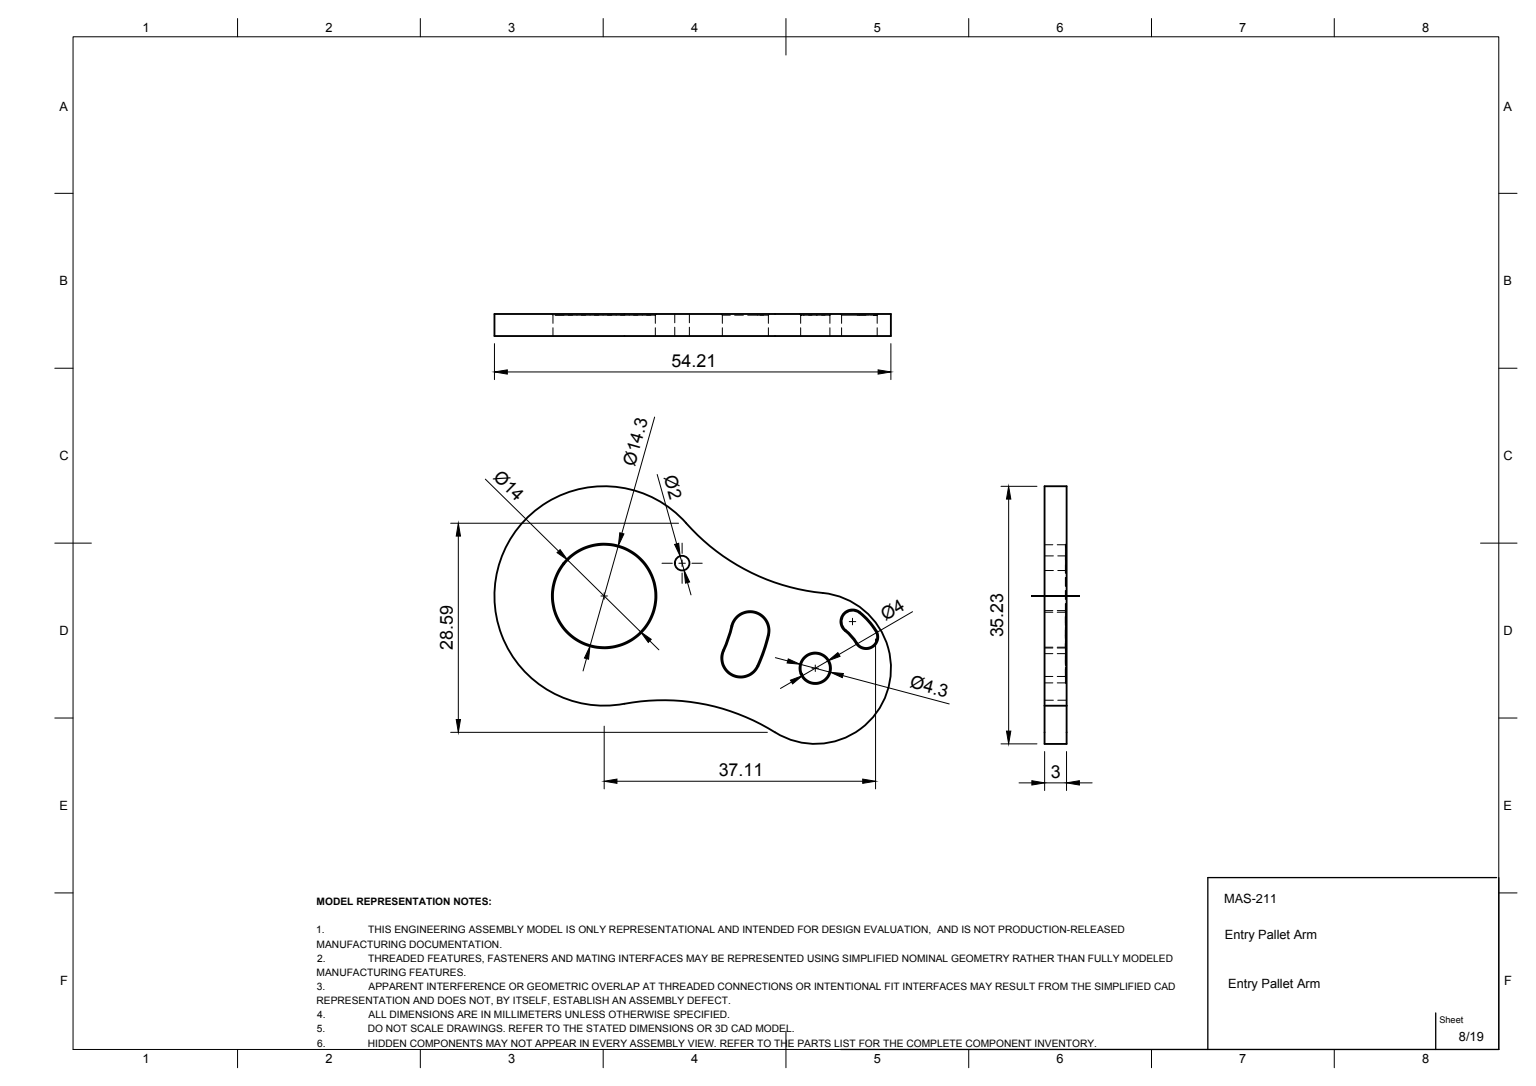
ISO-10303-21;
HEADER;
FILE_DESCRIPTION(
 (''),
 '2;1');
FILE_NAME ( 'Entry Pallet Arm.step', '2026-10-05T20:07:59+06:00', ( '' ), ( '' ), 'STEP AP214', 'Unspecified', '' );
FILE_SCHEMA (('AUTOMOTIVE_DESIGN { 1 0 10303 214 3 1 1 }'));
ENDSEC;
DATA;
#10=MECHANICAL_DESIGN_GEOMETRIC_PRESENTATION_REPRESENTATION('',(#325),#196741);
#131=ELLIPSE('',#8872,15.4840898363667,13.4083590367118) ;
#132=ELLIPSE('',#8873,20.0777465510975,17.3862071407653) ;
#133=ELLIPSE('',#8874,8.52758831083714,7.38294286669008) ;
#134=ELLIPSE('',#8875,5.66235728936404,4.9022943840305) ;
#325=STYLED_ITEM('',(#196765),#344) ;
#344=MANIFOLD_SOLID_BREP('Entry Pallet Arm',#8721) ;
#385=PLANE('',#8860) ;
#386=PLANE('',#8871) ;
#566=FACE_BOUND('',#1445,.T.) ;
#567=FACE_BOUND('',#1446,.T.) ;
#568=FACE_BOUND('',#1447,.T.) ;
#569=FACE_BOUND('',#1448,.T.) ;
#570=FACE_BOUND('',#1449,.T.) ;
#571=FACE_BOUND('',#1451,.T.) ;
#572=FACE_BOUND('',#1452,.T.) ;
#573=FACE_BOUND('',#1453,.T.) ;
#574=FACE_BOUND('',#1454,.T.) ;
#575=FACE_BOUND('',#1455,.T.) ;
#639=CIRCLE('',#8846,28.7407375552552) ;
#640=CIRCLE('',#8847,28.7407375552552) ;
#641=CIRCLE('',#8849,15.) ;
#642=CIRCLE('',#8850,15.) ;
#643=CIRCLE('',#8852,28.7407375552563) ;
#644=CIRCLE('',#8853,28.7407375552563) ;
#645=CIRCLE('',#8855,10.3432265401781) ;
#646=CIRCLE('',#8856,10.3432265401781) ;
#647=CIRCLE('',#8858,1.00000000000001) ;
#648=CIRCLE('',#8859,1.00000000000001) ;
#649=CIRCLE('',#8861,2.) ;
#650=CIRCLE('',#8862,23.0149881946395) ;
#651=CIRCLE('',#8863,2.4999999999999) ;
#652=CIRCLE('',#8864,18.0149881946822) ;
#653=CIRCLE('',#8865,2.49999999999983) ;
#654=CIRCLE('',#8866,7.00000000000001) ;
#655=CIRCLE('',#8867,1.50000000000001) ;
#656=CIRCLE('',#8868,6.6716132701064) ;
#657=CIRCLE('',#8869,1.49999999999977) ;
#658=CIRCLE('',#8870,9.6716132700902) ;
#659=CIRCLE('',#8877,2.00000000000002) ;
#660=CIRCLE('',#8880,18.0149881946813) ;
#661=CIRCLE('',#8884,7.00000000000001) ;
#662=CIRCLE('',#8887,1.49999999999978) ;
#663=CIRCLE('',#8889,6.6716132701049) ;
#836=B_SPLINE_SURFACE_WITH_KNOTS('',3,1,((#113116,#113117),(#113118,#113119),
(#113120,#113121),(#113122,#113123),(#113124,#113125),(#113126,#113127),
(#113128,#113129),(#113130,#113131),(#113132,#113133),(#113134,#113135),
(#113136,#113137),(#113138,#113139),(#113140,#113141),(#113142,#113143),
(#113144,#113145),(#113146,#113147),(#113148,#113149),(#113150,#113151),
(#113152,#113153)),.UNSPECIFIED.,.T.,.F.,.F.,(4,1,1,1,1,1,1,1,1,1,1,1,1,
1,1,1,4),(2,2),(0.,0.84428169467316,1.68856338934632,2.53284508400807,3.37712677866981,
4.22140847333581,5.06569016800181,5.90997186266355,6.75425355732529,7.5985352519836,
8.44281694664192,9.28709864130792,10.1313803359739,10.9756620306322,11.8199437252905,
12.664225419956,13.5085071146214),(-0.0112712723153948,0.214916064351503),
 .UNSPECIFIED.) ;
#837=B_SPLINE_SURFACE_WITH_KNOTS('',3,1,((#113155,#113156),(#113157,#113158),
(#113159,#113160),(#113161,#113162),(#113163,#113164),(#113165,#113166),
(#113167,#113168),(#113169,#113170),(#113171,#113172),(#113173,#113174),
(#113175,#113176)),.UNSPECIFIED.,.F.,.F.,.F.,(4,1,1,1,1,1,1,1,4),(2,2),
(0.,1.04064620349252,2.08129240698504,3.12193860703556,4.16258480708607,
5.2032310071414,6.24387720719673,7.28452341068926,8.32516961418179),(0.,
0.214915892336475),.UNSPECIFIED.) ;
#838=B_SPLINE_SURFACE_WITH_KNOTS('',3,1,((#113179,#113180),(#113181,#113182),
(#113183,#113184),(#113185,#113186)),.UNSPECIFIED.,.F.,.F.,.F.,(4,4),(2,
2),(-1.11022302462516E-16,3.4846841528001),(0.,0.212356567860224),
 .UNSPECIFIED.) ;
#839=B_SPLINE_SURFACE_WITH_KNOTS('',3,1,((#113188,#113189),(#113190,#113191),
(#113192,#113193),(#113194,#113195),(#113196,#113197),(#113198,#113199),
(#113200,#113201),(#113202,#113203),(#113204,#113205),(#113206,#113207),
(#113208,#113209)),.UNSPECIFIED.,.F.,.F.,.F.,(4,1,1,1,1,1,1,1,4),(2,2),
(0.,1.04062614942685,2.0812522988537,3.12187844827608,4.16250459769846,
5.20313074711661,6.24375689653477,7.28438304596783,8.32500919540089),(0.,
0.214916063344347),.UNSPECIFIED.) ;
#840=B_SPLINE_SURFACE_WITH_KNOTS('',3,1,((#113211,#113212),(#113213,#113214),
(#113215,#113216),(#113217,#113218)),.UNSPECIFIED.,.F.,.F.,.F.,(4,4),(2,
2),(1.11022302462516E-16,4.51848390029441),(-6.99189760998493E-5,0.212356567829038),
 .UNSPECIFIED.) ;
#841=B_SPLINE_SURFACE_WITH_KNOTS('',3,1,((#113219,#113220),(#113221,#113222),
(#113223,#113224),(#113225,#113226),(#113227,#113228),(#113229,#113230),
(#113231,#113232),(#113233,#113234),(#113235,#113236),(#113237,#113238),
(#113239,#113240),(#113241,#113242),(#113243,#113244),(#113245,#113246),
(#113247,#113248),(#113249,#113250),(#113251,#113252),(#113253,#113254),
(#113255,#113256)),.UNSPECIFIED.,.T.,.F.,.F.,(4,1,1,1,1,1,1,1,1,1,1,1,1,
1,1,1,4),(2,2),(0.,2.69519445779221,5.61545499238393,8.53571552697323,11.2309099847624,
13.9261044425515,16.8463649771433,19.7666255117326,22.4618199695218,25.1570144273109,
28.0772749619002,30.9975354964919,33.6927299542811,36.3879244120703,39.3081849466596,
42.2284454812513,44.9236399390405),(-0.021515064961137,0.21515064961137),
 .UNSPECIFIED.) ;
#842=B_SPLINE_SURFACE_WITH_KNOTS('',3,1,((#113258,#113259),(#113260,#113261),
(#113262,#113263),(#113264,#113265)),.UNSPECIFIED.,.F.,.F.,.F.,(4,4),(2,
2),(0.,3.40704145701401),(-0.000292126274588819,0.212844506430303),
 .UNSPECIFIED.) ;
#843=B_SPLINE_SURFACE_WITH_KNOTS('',3,1,((#113268,#113269),(#113270,#113271),
(#113272,#113273),(#113274,#113275),(#113276,#113277),(#113278,#113279),
(#113280,#113281),(#113282,#113283),(#113284,#113285)),.UNSPECIFIED.,.F.,
 .F.,.F.,(4,1,1,1,1,1,4),(2,2),(-0.00583358110187113,1.29587390932424,1.94381087119108,
2.59174783305793,3.23968479492214,3.88762175678635,5.18932922796654),(-0.00583356183498457,
0.218727515757821),.UNSPECIFIED.) ;
#844=B_SPLINE_SURFACE_WITH_KNOTS('',3,1,((#113287,#113288),(#113289,#113290),
(#113291,#113292),(#113293,#113294)),.UNSPECIFIED.,.F.,.F.,.F.,(4,4),(2,
2),(0.,2.26229870547718),(0.,0.212844507129699),.UNSPECIFIED.) ;
#845=B_SPLINE_SURFACE_WITH_KNOTS('',3,1,((#113296,#113297),(#113298,#113299),
(#113300,#113301),(#113302,#113303),(#113304,#113305),(#113306,#113307),
(#113308,#113309),(#113310,#113311),(#113312,#113313)),.UNSPECIFIED.,.F.,
 .F.,.F.,(4,1,1,1,1,1,4),(2,2),(0.,1.29587422179682,1.94381133989722,2.59174845799762,
3.23968557610065,3.88762269420369,5.18349660704779),(0.,0.218727518540508),
 .UNSPECIFIED.) ;
#954=FACE_OUTER_BOUND('',#1439,.T.) ;
#955=FACE_OUTER_BOUND('',#1440,.T.) ;
#956=FACE_OUTER_BOUND('',#1441,.T.) ;
#957=FACE_OUTER_BOUND('',#1442,.T.) ;
#958=FACE_OUTER_BOUND('',#1443,.T.) ;
#959=FACE_OUTER_BOUND('',#1444,.T.) ;
#960=FACE_OUTER_BOUND('',#1450,.T.) ;
#961=FACE_OUTER_BOUND('',#1456,.T.) ;
#962=FACE_OUTER_BOUND('',#1457,.T.) ;
#963=FACE_OUTER_BOUND('',#1458,.T.) ;
#964=FACE_OUTER_BOUND('',#1459,.T.) ;
#965=FACE_OUTER_BOUND('',#1460,.T.) ;
#966=FACE_OUTER_BOUND('',#1461,.T.) ;
#967=FACE_OUTER_BOUND('',#1462,.T.) ;
#968=FACE_OUTER_BOUND('',#1463,.T.) ;
#969=FACE_OUTER_BOUND('',#1464,.T.) ;
#970=FACE_OUTER_BOUND('',#1465,.T.) ;
#971=FACE_OUTER_BOUND('',#1466,.T.) ;
#972=FACE_OUTER_BOUND('',#1467,.T.) ;
#973=FACE_OUTER_BOUND('',#1468,.T.) ;
#974=FACE_OUTER_BOUND('',#1469,.T.) ;
#975=FACE_OUTER_BOUND('',#1470,.T.) ;
#976=FACE_OUTER_BOUND('',#1471,.T.) ;
#977=FACE_OUTER_BOUND('',#1472,.T.) ;
#978=FACE_OUTER_BOUND('',#1473,.T.) ;
#979=FACE_OUTER_BOUND('',#1474,.T.) ;
#980=FACE_OUTER_BOUND('',#1475,.T.) ;
#1439=EDGE_LOOP('',(#6086,#6087,#6088,#6089)) ;
#1440=EDGE_LOOP('',(#6090,#6091,#6092,#6093)) ;
#1441=EDGE_LOOP('',(#6094,#6095,#6096,#6097)) ;
#1442=EDGE_LOOP('',(#6098,#6099,#6100,#6101)) ;
#1443=EDGE_LOOP('',(#6102,#6103,#6104,#6105)) ;
#1444=EDGE_LOOP('',(#6106,#6107,#6108,#6109)) ;
#1445=EDGE_LOOP('',(#6110)) ;
#1446=EDGE_LOOP('',(#6111,#6112,#6113,#6114)) ;
#1447=EDGE_LOOP('',(#6115)) ;
#1448=EDGE_LOOP('',(#6116,#6117,#6118,#6119)) ;
#1449=EDGE_LOOP('',(#6120)) ;
#1450=EDGE_LOOP('',(#6121,#6122,#6123,#6124)) ;
#1451=EDGE_LOOP('',(#6125)) ;
#1452=EDGE_LOOP('',(#6126)) ;
#1453=EDGE_LOOP('',(#6127,#6128,#6129,#6130)) ;
#1454=EDGE_LOOP('',(#6131,#6132,#6133,#6134)) ;
#1455=EDGE_LOOP('',(#6135)) ;
#1456=EDGE_LOOP('',(#6136,#6137,#6138,#6139)) ;
#1457=EDGE_LOOP('',(#6140,#6141,#6142,#6143)) ;
#1458=EDGE_LOOP('',(#6144,#6145,#6146,#6147)) ;
#1459=EDGE_LOOP('',(#6148,#6149,#6150,#6151)) ;
#1460=EDGE_LOOP('',(#6152,#6153,#6154,#6155)) ;
#1461=EDGE_LOOP('',(#6156,#6157,#6158,#6159)) ;
#1462=EDGE_LOOP('',(#6160,#6161,#6162,#6163)) ;
#1463=EDGE_LOOP('',(#6164,#6165,#6166,#6167)) ;
#1464=EDGE_LOOP('',(#6168,#6169,#6170,#6171)) ;
#1465=EDGE_LOOP('',(#6172,#6173,#6174,#6175)) ;
#1466=EDGE_LOOP('',(#6176,#6177,#6178,#6179)) ;
#1467=EDGE_LOOP('',(#6180,#6181,#6182,#6183)) ;
#1468=EDGE_LOOP('',(#6184,#6185,#6186,#6187)) ;
#1469=EDGE_LOOP('',(#6188,#6189,#6190,#6191)) ;
#1470=EDGE_LOOP('',(#6192,#6193,#6194,#6195)) ;
#1471=EDGE_LOOP('',(#6196,#6197,#6198,#6199)) ;
#1472=EDGE_LOOP('',(#6200,#6201,#6202,#6203)) ;
#1473=EDGE_LOOP('',(#6204,#6205,#6206,#6207)) ;
#1474=EDGE_LOOP('',(#6208,#6209,#6210,#6211)) ;
#1475=EDGE_LOOP('',(#6212,#6213,#6214,#6215)) ;
#1956=LINE('',#112886,#2659) ;
#1957=LINE('',#112889,#2660) ;
#1958=LINE('',#112894,#2661) ;
#1959=LINE('',#112900,#2662) ;
#1960=LINE('',#112909,#2663) ;
#1961=LINE('',#113041,#2664) ;
#1962=LINE('',#113044,#2665) ;
#1963=LINE('',#113046,#2666) ;
#1964=LINE('',#113060,#2667) ;
#1965=LINE('',#113064,#2668) ;
#1966=LINE('',#113086,#2669) ;
#1967=LINE('',#113089,#2670) ;
#1968=LINE('',#113091,#2671) ;
#1969=LINE('',#113100,#2672) ;
#1970=LINE('',#113104,#2673) ;
#1971=LINE('',#113154,#2674) ;
#1972=LINE('',#113177,#2675) ;
#1973=LINE('',#113178,#2676) ;
#1974=LINE('',#113187,#2677) ;
#1975=LINE('',#113210,#2678) ;
#1976=LINE('',#113257,#2679) ;
#1977=LINE('',#113266,#2680) ;
#1978=LINE('',#113267,#2681) ;
#1979=LINE('',#113286,#2682) ;
#1980=LINE('',#113295,#2683) ;
#2659=VECTOR('',#9750,10.) ;
#2660=VECTOR('',#9753,10.) ;
#2661=VECTOR('',#9758,10.) ;
#2662=VECTOR('',#9765,10.) ;
#2663=VECTOR('',#9778,1.00000000000001) ;
#2664=VECTOR('',#9817,2.00000000000002) ;
#2665=VECTOR('',#9820,10.) ;
#2666=VECTOR('',#9821,10.) ;
#2667=VECTOR('',#9824,10.) ;
#2668=VECTOR('',#9829,10.) ;
#2669=VECTOR('',#9836,6.99999999999997) ;
#2670=VECTOR('',#9839,10.) ;
#2671=VECTOR('',#9840,10.) ;
#2672=VECTOR('',#9843,10.) ;
#2673=VECTOR('',#9848,10.) ;
#2674=VECTOR('',#9853,10.) ;
#2675=VECTOR('',#9854,10.) ;
#2676=VECTOR('',#9855,10.) ;
#2677=VECTOR('',#9856,10.) ;
#2678=VECTOR('',#9857,10.) ;
#2679=VECTOR('',#9858,10.) ;
#2680=VECTOR('',#9859,10.) ;
#2681=VECTOR('',#9860,10.) ;
#2682=VECTOR('',#9861,10.) ;
#2683=VECTOR('',#9862,10.) ;
#3408=B_SPLINE_CURVE_WITH_KNOTS('',3,(#112934,#112935,#112936,#112937,#112938,
#112939,#112940,#112941,#112942,#112943,#112944,#112945,#112946,#112947,
#112948,#112949,#112950,#112951,#112952),.UNSPECIFIED.,.T.,.F.,(4,1,1,1,
1,1,1,1,1,1,1,1,1,1,1,1,4),(0.,2.69519445779221,5.61545499238393,8.53571552697323,
11.2309099847624,13.9261044425515,16.8463649771433,19.7666255117326,22.4618199695218,
25.1570144273109,28.0772749619002,30.9975354964919,33.6927299542811,36.3879244120703,
39.3081849466596,42.2284454812513,44.9236399390405),.UNSPECIFIED.) ;
#3409=B_SPLINE_CURVE_WITH_KNOTS('',3,(#112955,#112956,#112957,#112958,#112959,
#112960,#112961,#112962,#112963,#112964,#112965),.UNSPECIFIED.,.F.,.F.,
(4,1,1,1,1,1,1,1,4),(0.,1.04064620349252,2.08129240698504,3.12193860703556,
4.16258480708607,5.2032310071414,6.24387720719673,7.28452341068926,8.32516961418179),
 .UNSPECIFIED.) ;
#3410=B_SPLINE_CURVE_WITH_KNOTS('',3,(#112969,#112970,#112971,#112972,#112973,
#112974,#112975,#112976,#112977,#112978,#112979),.UNSPECIFIED.,.F.,.F.,
(4,1,1,1,1,1,1,1,4),(0.,1.04062614942685,2.0812522988537,3.12187844827608,
4.16250459769846,5.20313074711661,6.24375689653477,7.28438304596783,8.32500919540089),
 .UNSPECIFIED.) ;
#3411=B_SPLINE_CURVE_WITH_KNOTS('',3,(#112985,#112986,#112987,#112988,#112989,
#112990,#112991,#112992,#112993,#112994,#112995,#112996,#112997,#112998,
#112999,#113000,#113001,#113002,#113003,#113004,#113005,#113006),
 .UNSPECIFIED.,.F.,.F.,(4,2,2,2,2,2,2,2,2,2,4),(-0.482562577818028,-0.447777673419887,
-0.413036999106612,-0.354121907354326,-0.297189647078672,-0.24122658651999,
-0.185260249381691,-0.128411301285868,-0.0694119365245573,-0.0347286016619977,
0.),.UNSPECIFIED.) ;
#3412=B_SPLINE_CURVE_WITH_KNOTS('',3,(#113009,#113010,#113011,#113012,#113013,
#113014,#113015,#113016,#113017),.UNSPECIFIED.,.F.,.F.,(4,1,1,1,1,1,4),
(0.,1.29587422179682,1.94381133989722,2.59174845799762,3.23968557610065,
3.88762269420369,5.18349660704779),.UNSPECIFIED.) ;
#3413=B_SPLINE_CURVE_WITH_KNOTS('',3,(#113019,#113020,#113021,#113022,#113023,
#113024,#113025,#113026,#113027,#113028,#113029,#113030,#113031,#113032,
#113033,#113034,#113035,#113036,#113037),.UNSPECIFIED.,.T.,.F.,(4,1,1,1,
1,1,1,1,1,1,1,1,1,1,1,1,4),(0.,0.84428169467316,1.68856338934632,2.53284508400807,
3.37712677866981,4.22140847333581,5.06569016800181,5.90997186266355,6.75425355732529,
7.5985352519836,8.44281694664192,9.28709864130792,10.1313803359739,10.9756620306322,
11.8199437252905,12.664225419956,13.5085071146214),.UNSPECIFIED.) ;
#3414=B_SPLINE_CURVE_WITH_KNOTS('',3,(#113047,#113048,#113049,#113050,#113051,
#113052,#113053,#113054,#113055,#113056,#113057),.UNSPECIFIED.,.F.,.F.,
(4,1,1,1,1,1,1,1,4),(0.,1.04064620349252,2.08129240698504,3.12193860703556,
4.16258480708607,5.2032310071414,6.24387720719673,7.28452341068926,8.32516961418179),
 .UNSPECIFIED.) ;
#3415=B_SPLINE_CURVE_WITH_KNOTS('',3,(#113065,#113066,#113067,#113068,#113069,
#113070,#113071,#113072,#113073,#113074,#113075),.UNSPECIFIED.,.F.,.F.,
(4,1,1,1,1,1,1,1,4),(0.,1.04062614942685,2.0812522988537,3.12187844827608,
4.16250459769846,5.20313074711661,6.24375689653477,7.28438304596783,8.32500919540089),
 .UNSPECIFIED.) ;
#3416=B_SPLINE_CURVE_WITH_KNOTS('',3,(#113077,#113078,#113079,#113080,#113081,
#113082),.UNSPECIFIED.,.F.,.F.,(4,2,4),(0.,0.224505556318787,0.44901111263762),
 .UNSPECIFIED.) ;
#3417=B_SPLINE_CURVE_WITH_KNOTS('',3,(#113092,#113093,#113094,#113095,#113096,
#113097),.UNSPECIFIED.,.F.,.F.,(4,2,4),(6.6871801508411E-9,0.167853757777579,
0.335707403334044),.UNSPECIFIED.) ;
#3418=B_SPLINE_CURVE_WITH_KNOTS('',3,(#113107,#113108,#113109,#113110,#113111,
#113112,#113113,#113114,#113115),.UNSPECIFIED.,.F.,.F.,(4,1,1,1,1,1,4),
(1.11022302462516E-16,1.29587422179682,1.94381133989722,2.59174845799762,
3.23968557610065,3.88762269420369,5.18349660704779),.UNSPECIFIED.) ;
#3623=VERTEX_POINT('',#112882) ;
#3624=VERTEX_POINT('',#112883) ;
#3625=VERTEX_POINT('',#112885) ;
#3626=VERTEX_POINT('',#112887) ;
#3627=VERTEX_POINT('',#112891) ;
#3628=VERTEX_POINT('',#112893) ;
#3629=VERTEX_POINT('',#112897) ;
#3630=VERTEX_POINT('',#112899) ;
#3631=VERTEX_POINT('',#112906) ;
#3632=VERTEX_POINT('',#112908) ;
#3633=VERTEX_POINT('',#112912) ;
#3634=VERTEX_POINT('',#112914) ;
#3635=VERTEX_POINT('',#112915) ;
#3636=VERTEX_POINT('',#112917) ;
#3637=VERTEX_POINT('',#112919) ;
#3638=VERTEX_POINT('',#112922) ;
#3639=VERTEX_POINT('',#112924) ;
#3640=VERTEX_POINT('',#112925) ;
#3641=VERTEX_POINT('',#112927) ;
#3642=VERTEX_POINT('',#112929) ;
#3643=VERTEX_POINT('',#112933) ;
#3644=VERTEX_POINT('',#112953) ;
#3645=VERTEX_POINT('',#112954) ;
#3646=VERTEX_POINT('',#112966) ;
#3647=VERTEX_POINT('',#112968) ;
#3648=VERTEX_POINT('',#112981) ;
#3649=VERTEX_POINT('',#112982) ;
#3650=VERTEX_POINT('',#112984) ;
#3651=VERTEX_POINT('',#113007) ;
#3652=VERTEX_POINT('',#113018) ;
#3653=VERTEX_POINT('',#113039) ;
#3654=VERTEX_POINT('',#113043) ;
#3655=VERTEX_POINT('',#113045) ;
#3656=VERTEX_POINT('',#113059) ;
#3657=VERTEX_POINT('',#113063) ;
#3658=VERTEX_POINT('',#113084) ;
#3659=VERTEX_POINT('',#113088) ;
#3660=VERTEX_POINT('',#113090) ;
#3661=VERTEX_POINT('',#113099) ;
#3662=VERTEX_POINT('',#113103) ;
#4551=EDGE_CURVE('',#3623,#3624,#639,.T.) ;
#4552=EDGE_CURVE('',#3624,#3625,#1956,.T.) ;
#4553=EDGE_CURVE('',#3626,#3625,#640,.T.) ;
#4554=EDGE_CURVE('',#3623,#3626,#1957,.T.) ;
#4555=EDGE_CURVE('',#3624,#3627,#641,.T.) ;
#4556=EDGE_CURVE('',#3627,#3628,#1958,.T.) ;
#4557=EDGE_CURVE('',#3625,#3628,#642,.T.) ;
#4558=EDGE_CURVE('',#3627,#3629,#643,.T.) ;
#4559=EDGE_CURVE('',#3629,#3630,#1959,.T.) ;
#4560=EDGE_CURVE('',#3628,#3630,#644,.T.) ;
#4561=EDGE_CURVE('',#3629,#3623,#645,.T.) ;
#4562=EDGE_CURVE('',#3630,#3626,#646,.T.) ;
#4563=EDGE_CURVE('',#3631,#3631,#647,.T.) ;
#4564=EDGE_CURVE('',#3631,#3632,#1960,.T.) ;
#4565=EDGE_CURVE('',#3632,#3632,#648,.T.) ;
#4566=EDGE_CURVE('',#3633,#3633,#649,.T.) ;
#4567=EDGE_CURVE('',#3634,#3635,#650,.T.) ;
#4568=EDGE_CURVE('',#3636,#3634,#651,.T.) ;
#4569=EDGE_CURVE('',#3637,#3636,#652,.T.) ;
#4570=EDGE_CURVE('',#3635,#3637,#653,.T.) ;
#4571=EDGE_CURVE('',#3638,#3638,#654,.T.) ;
#4572=EDGE_CURVE('',#3639,#3640,#655,.T.) ;
#4573=EDGE_CURVE('',#3641,#3639,#656,.T.) ;
#4574=EDGE_CURVE('',#3642,#3641,#657,.T.) ;
#4575=EDGE_CURVE('',#3640,#3642,#658,.T.) ;
#4576=EDGE_CURVE('',#3643,#3643,#3408,.T.) ;
#4577=EDGE_CURVE('',#3644,#3645,#3409,.T.) ;
#4578=EDGE_CURVE('',#3645,#3646,#131,.T.) ;
#4579=EDGE_CURVE('',#3646,#3647,#3410,.T.) ;
#4580=EDGE_CURVE('',#3647,#3644,#132,.T.) ;
#4581=EDGE_CURVE('',#3648,#3649,#133,.T.) ;
#4582=EDGE_CURVE('',#3649,#3650,#3411,.T.) ;
#4583=EDGE_CURVE('',#3650,#3651,#134,.T.) ;
#4584=EDGE_CURVE('',#3651,#3648,#3412,.T.) ;
#4585=EDGE_CURVE('',#3652,#3652,#3413,.T.) ;
#4586=EDGE_CURVE('',#3653,#3653,#659,.T.) ;
#4587=EDGE_CURVE('',#3653,#3633,#1961,.T.) ;
#4588=EDGE_CURVE('',#3635,#3654,#1962,.T.) ;
#4589=EDGE_CURVE('',#3637,#3655,#1963,.T.) ;
#4590=EDGE_CURVE('',#3654,#3655,#3414,.T.) ;
#4591=EDGE_CURVE('',#3636,#3656,#1964,.T.) ;
#4592=EDGE_CURVE('',#3655,#3656,#660,.T.) ;
#4593=EDGE_CURVE('',#3634,#3657,#1965,.T.) ;
#4594=EDGE_CURVE('',#3656,#3657,#3415,.T.) ;
#4595=EDGE_CURVE('',#3657,#3654,#3416,.T.) ;
#4596=EDGE_CURVE('',#3658,#3658,#661,.T.) ;
#4597=EDGE_CURVE('',#3658,#3638,#1966,.T.) ;
#4598=EDGE_CURVE('',#3640,#3659,#1967,.T.) ;
#4599=EDGE_CURVE('',#3642,#3660,#1968,.T.) ;
#4600=EDGE_CURVE('',#3659,#3660,#3417,.T.) ;
#4601=EDGE_CURVE('',#3641,#3661,#1969,.T.) ;
#4602=EDGE_CURVE('',#3660,#3661,#662,.T.) ;
#4603=EDGE_CURVE('',#3639,#3662,#1970,.T.) ;
#4604=EDGE_CURVE('',#3661,#3662,#663,.T.) ;
#4605=EDGE_CURVE('',#3662,#3659,#3418,.T.) ;
#4606=EDGE_CURVE('',#3653,#3652,#1971,.T.) ;
#4607=EDGE_CURVE('',#3655,#3645,#1972,.T.) ;
#4608=EDGE_CURVE('',#3644,#3654,#1973,.T.) ;
#4609=EDGE_CURVE('',#3646,#3656,#1974,.T.) ;
#4610=EDGE_CURVE('',#3657,#3647,#1975,.T.) ;
#4611=EDGE_CURVE('',#3658,#3643,#1976,.T.) ;
#4612=EDGE_CURVE('',#3660,#3649,#1977,.T.) ;
#4613=EDGE_CURVE('',#3648,#3659,#1978,.T.) ;
#4614=EDGE_CURVE('',#3661,#3650,#1979,.T.) ;
#4615=EDGE_CURVE('',#3651,#3662,#1980,.T.) ;
#6086=ORIENTED_EDGE('',*,*,#4551,.T.) ;
#6087=ORIENTED_EDGE('',*,*,#4552,.T.) ;
#6088=ORIENTED_EDGE('',*,*,#4553,.F.) ;
#6089=ORIENTED_EDGE('',*,*,#4554,.F.) ;
#6090=ORIENTED_EDGE('',*,*,#4555,.T.) ;
#6091=ORIENTED_EDGE('',*,*,#4556,.T.) ;
#6092=ORIENTED_EDGE('',*,*,#4557,.F.) ;
#6093=ORIENTED_EDGE('',*,*,#4552,.F.) ;
#6094=ORIENTED_EDGE('',*,*,#4558,.T.) ;
#6095=ORIENTED_EDGE('',*,*,#4559,.T.) ;
#6096=ORIENTED_EDGE('',*,*,#4560,.F.) ;
#6097=ORIENTED_EDGE('',*,*,#4556,.F.) ;
#6098=ORIENTED_EDGE('',*,*,#4561,.T.) ;
#6099=ORIENTED_EDGE('',*,*,#4554,.T.) ;
#6100=ORIENTED_EDGE('',*,*,#4562,.F.) ;
#6101=ORIENTED_EDGE('',*,*,#4559,.F.) ;
#6102=ORIENTED_EDGE('',*,*,#4563,.F.) ;
#6103=ORIENTED_EDGE('',*,*,#4564,.T.) ;
#6104=ORIENTED_EDGE('',*,*,#4565,.T.) ;
#6105=ORIENTED_EDGE('',*,*,#4564,.F.) ;
#6106=ORIENTED_EDGE('',*,*,#4561,.F.) ;
#6107=ORIENTED_EDGE('',*,*,#4558,.F.) ;
#6108=ORIENTED_EDGE('',*,*,#4555,.F.) ;
#6109=ORIENTED_EDGE('',*,*,#4551,.F.) ;
#6110=ORIENTED_EDGE('',*,*,#4566,.F.) ;
#6111=ORIENTED_EDGE('',*,*,#4567,.F.) ;
#6112=ORIENTED_EDGE('',*,*,#4568,.F.) ;
#6113=ORIENTED_EDGE('',*,*,#4569,.F.) ;
#6114=ORIENTED_EDGE('',*,*,#4570,.F.) ;
#6115=ORIENTED_EDGE('',*,*,#4571,.F.) ;
#6116=ORIENTED_EDGE('',*,*,#4572,.F.) ;
#6117=ORIENTED_EDGE('',*,*,#4573,.F.) ;
#6118=ORIENTED_EDGE('',*,*,#4574,.F.) ;
#6119=ORIENTED_EDGE('',*,*,#4575,.F.) ;
#6120=ORIENTED_EDGE('',*,*,#4565,.F.) ;
#6121=ORIENTED_EDGE('',*,*,#4553,.T.) ;
#6122=ORIENTED_EDGE('',*,*,#4557,.T.) ;
#6123=ORIENTED_EDGE('',*,*,#4560,.T.) ;
#6124=ORIENTED_EDGE('',*,*,#4562,.T.) ;
#6125=ORIENTED_EDGE('',*,*,#4563,.T.) ;
#6126=ORIENTED_EDGE('',*,*,#4576,.T.) ;
#6127=ORIENTED_EDGE('',*,*,#4577,.T.) ;
#6128=ORIENTED_EDGE('',*,*,#4578,.T.) ;
#6129=ORIENTED_EDGE('',*,*,#4579,.T.) ;
#6130=ORIENTED_EDGE('',*,*,#4580,.T.) ;
#6131=ORIENTED_EDGE('',*,*,#4581,.T.) ;
#6132=ORIENTED_EDGE('',*,*,#4582,.T.) ;
#6133=ORIENTED_EDGE('',*,*,#4583,.T.) ;
#6134=ORIENTED_EDGE('',*,*,#4584,.T.) ;
#6135=ORIENTED_EDGE('',*,*,#4585,.T.) ;
#6136=ORIENTED_EDGE('',*,*,#4586,.F.) ;
#6137=ORIENTED_EDGE('',*,*,#4587,.T.) ;
#6138=ORIENTED_EDGE('',*,*,#4566,.T.) ;
#6139=ORIENTED_EDGE('',*,*,#4587,.F.) ;
#6140=ORIENTED_EDGE('',*,*,#4588,.F.) ;
#6141=ORIENTED_EDGE('',*,*,#4570,.T.) ;
#6142=ORIENTED_EDGE('',*,*,#4589,.T.) ;
#6143=ORIENTED_EDGE('',*,*,#4590,.F.) ;
#6144=ORIENTED_EDGE('',*,*,#4589,.F.) ;
#6145=ORIENTED_EDGE('',*,*,#4569,.T.) ;
#6146=ORIENTED_EDGE('',*,*,#4591,.T.) ;
#6147=ORIENTED_EDGE('',*,*,#4592,.F.) ;
#6148=ORIENTED_EDGE('',*,*,#4591,.F.) ;
#6149=ORIENTED_EDGE('',*,*,#4568,.T.) ;
#6150=ORIENTED_EDGE('',*,*,#4593,.T.) ;
#6151=ORIENTED_EDGE('',*,*,#4594,.F.) ;
#6152=ORIENTED_EDGE('',*,*,#4593,.F.) ;
#6153=ORIENTED_EDGE('',*,*,#4567,.T.) ;
#6154=ORIENTED_EDGE('',*,*,#4588,.T.) ;
#6155=ORIENTED_EDGE('',*,*,#4595,.F.) ;
#6156=ORIENTED_EDGE('',*,*,#4596,.F.) ;
#6157=ORIENTED_EDGE('',*,*,#4597,.T.) ;
#6158=ORIENTED_EDGE('',*,*,#4571,.T.) ;
#6159=ORIENTED_EDGE('',*,*,#4597,.F.) ;
#6160=ORIENTED_EDGE('',*,*,#4598,.F.) ;
#6161=ORIENTED_EDGE('',*,*,#4575,.T.) ;
#6162=ORIENTED_EDGE('',*,*,#4599,.T.) ;
#6163=ORIENTED_EDGE('',*,*,#4600,.F.) ;
#6164=ORIENTED_EDGE('',*,*,#4599,.F.) ;
#6165=ORIENTED_EDGE('',*,*,#4574,.T.) ;
#6166=ORIENTED_EDGE('',*,*,#4601,.T.) ;
#6167=ORIENTED_EDGE('',*,*,#4602,.F.) ;
#6168=ORIENTED_EDGE('',*,*,#4601,.F.) ;
#6169=ORIENTED_EDGE('',*,*,#4573,.T.) ;
#6170=ORIENTED_EDGE('',*,*,#4603,.T.) ;
#6171=ORIENTED_EDGE('',*,*,#4604,.F.) ;
#6172=ORIENTED_EDGE('',*,*,#4603,.F.) ;
#6173=ORIENTED_EDGE('',*,*,#4572,.T.) ;
#6174=ORIENTED_EDGE('',*,*,#4598,.T.) ;
#6175=ORIENTED_EDGE('',*,*,#4605,.F.) ;
#6176=ORIENTED_EDGE('',*,*,#4586,.T.) ;
#6177=ORIENTED_EDGE('',*,*,#4606,.T.) ;
#6178=ORIENTED_EDGE('',*,*,#4585,.F.) ;
#6179=ORIENTED_EDGE('',*,*,#4606,.F.) ;
#6180=ORIENTED_EDGE('',*,*,#4590,.T.) ;
#6181=ORIENTED_EDGE('',*,*,#4607,.T.) ;
#6182=ORIENTED_EDGE('',*,*,#4577,.F.) ;
#6183=ORIENTED_EDGE('',*,*,#4608,.T.) ;
#6184=ORIENTED_EDGE('',*,*,#4592,.T.) ;
#6185=ORIENTED_EDGE('',*,*,#4609,.F.) ;
#6186=ORIENTED_EDGE('',*,*,#4578,.F.) ;
#6187=ORIENTED_EDGE('',*,*,#4607,.F.) ;
#6188=ORIENTED_EDGE('',*,*,#4594,.T.) ;
#6189=ORIENTED_EDGE('',*,*,#4610,.T.) ;
#6190=ORIENTED_EDGE('',*,*,#4579,.F.) ;
#6191=ORIENTED_EDGE('',*,*,#4609,.T.) ;
#6192=ORIENTED_EDGE('',*,*,#4595,.T.) ;
#6193=ORIENTED_EDGE('',*,*,#4608,.F.) ;
#6194=ORIENTED_EDGE('',*,*,#4580,.F.) ;
#6195=ORIENTED_EDGE('',*,*,#4610,.F.) ;
#6196=ORIENTED_EDGE('',*,*,#4596,.T.) ;
#6197=ORIENTED_EDGE('',*,*,#4611,.T.) ;
#6198=ORIENTED_EDGE('',*,*,#4576,.F.) ;
#6199=ORIENTED_EDGE('',*,*,#4611,.F.) ;
#6200=ORIENTED_EDGE('',*,*,#4600,.T.) ;
#6201=ORIENTED_EDGE('',*,*,#4612,.T.) ;
#6202=ORIENTED_EDGE('',*,*,#4581,.F.) ;
#6203=ORIENTED_EDGE('',*,*,#4613,.T.) ;
#6204=ORIENTED_EDGE('',*,*,#4602,.T.) ;
#6205=ORIENTED_EDGE('',*,*,#4614,.T.) ;
#6206=ORIENTED_EDGE('',*,*,#4582,.F.) ;
#6207=ORIENTED_EDGE('',*,*,#4612,.F.) ;
#6208=ORIENTED_EDGE('',*,*,#4604,.T.) ;
#6209=ORIENTED_EDGE('',*,*,#4615,.F.) ;
#6210=ORIENTED_EDGE('',*,*,#4583,.F.) ;
#6211=ORIENTED_EDGE('',*,*,#4614,.F.) ;
#6212=ORIENTED_EDGE('',*,*,#4605,.T.) ;
#6213=ORIENTED_EDGE('',*,*,#4613,.F.) ;
#6214=ORIENTED_EDGE('',*,*,#4584,.F.) ;
#6215=ORIENTED_EDGE('',*,*,#4615,.T.) ;
#8154=CYLINDRICAL_SURFACE('',#8845,28.7407375552551) ;
#8155=CYLINDRICAL_SURFACE('',#8848,15.) ;
#8156=CYLINDRICAL_SURFACE('',#8851,28.7407375552569) ;
#8157=CYLINDRICAL_SURFACE('',#8854,10.3432265401782) ;
#8158=CYLINDRICAL_SURFACE('',#8857,1.00000000000001) ;
#8159=CYLINDRICAL_SURFACE('',#8876,2.00000000000002) ;
#8160=CYLINDRICAL_SURFACE('',#8878,2.4999999999999) ;
#8161=CYLINDRICAL_SURFACE('',#8879,18.0149881946833) ;
#8162=CYLINDRICAL_SURFACE('',#8881,2.49999999999991) ;
#8163=CYLINDRICAL_SURFACE('',#8882,23.0149881946373) ;
#8164=CYLINDRICAL_SURFACE('',#8883,6.99999999999997) ;
#8165=CYLINDRICAL_SURFACE('',#8885,9.6716132700902) ;
#8166=CYLINDRICAL_SURFACE('',#8886,1.49999999999984) ;
#8167=CYLINDRICAL_SURFACE('',#8888,6.67161327010488) ;
#8168=CYLINDRICAL_SURFACE('',#8890,1.50000000000001) ;
#8337=ADVANCED_FACE('',(#954),#8154,.F.) ;
#8338=ADVANCED_FACE('',(#955),#8155,.T.) ;
#8339=ADVANCED_FACE('',(#956),#8156,.F.) ;
#8340=ADVANCED_FACE('',(#957),#8157,.T.) ;
#8341=ADVANCED_FACE('',(#958),#8158,.F.) ;
#8342=ADVANCED_FACE('',(#959,#566,#567,#568,#569,#570),#385,.T.) ;
#8343=ADVANCED_FACE('',(#960,#571,#572,#573,#574,#575),#386,.T.) ;
#8344=ADVANCED_FACE('',(#961),#8159,.F.) ;
#8345=ADVANCED_FACE('',(#962),#8160,.F.) ;
#8346=ADVANCED_FACE('',(#963),#8161,.T.) ;
#8347=ADVANCED_FACE('',(#964),#8162,.F.) ;
#8348=ADVANCED_FACE('',(#965),#8163,.F.) ;
#8349=ADVANCED_FACE('',(#966),#8164,.F.) ;
#8350=ADVANCED_FACE('',(#967),#8165,.F.) ;
#8351=ADVANCED_FACE('',(#968),#8166,.F.) ;
#8352=ADVANCED_FACE('',(#969),#8167,.T.) ;
#8353=ADVANCED_FACE('',(#970),#8168,.F.) ;
#8354=ADVANCED_FACE('',(#971),#836,.T.) ;
#8355=ADVANCED_FACE('',(#972),#837,.T.) ;
#8356=ADVANCED_FACE('',(#973),#838,.T.) ;
#8357=ADVANCED_FACE('',(#974),#839,.T.) ;
#8358=ADVANCED_FACE('',(#975),#840,.T.) ;
#8359=ADVANCED_FACE('',(#976),#841,.T.) ;
#8360=ADVANCED_FACE('',(#977),#842,.T.) ;
#8361=ADVANCED_FACE('',(#978),#843,.T.) ;
#8362=ADVANCED_FACE('',(#979),#844,.T.) ;
#8363=ADVANCED_FACE('',(#980),#845,.T.) ;
#8721=CLOSED_SHELL('',(#8337,#8338,#8339,#8340,#8341,#8342,#8343,#8344,
#8345,#8346,#8347,#8348,#8349,#8350,#8351,#8352,#8353,#8354,#8355,#8356,
#8357,#8358,#8359,#8360,#8361,#8362,#8363)) ;
#8845=AXIS2_PLACEMENT_3D('',#112881,#9746,#9747) ;
#8846=AXIS2_PLACEMENT_3D('',#112884,#9748,#9749) ;
#8847=AXIS2_PLACEMENT_3D('',#112888,#9751,#9752) ;
#8848=AXIS2_PLACEMENT_3D('',#112890,#9754,#9755) ;
#8849=AXIS2_PLACEMENT_3D('',#112892,#9756,#9757) ;
#8850=AXIS2_PLACEMENT_3D('',#112895,#9759,#9760) ;
#8851=AXIS2_PLACEMENT_3D('',#112896,#9761,#9762) ;
#8852=AXIS2_PLACEMENT_3D('',#112898,#9763,#9764) ;
#8853=AXIS2_PLACEMENT_3D('',#112901,#9766,#9767) ;
#8854=AXIS2_PLACEMENT_3D('',#112902,#9768,#9769) ;
#8855=AXIS2_PLACEMENT_3D('',#112903,#9770,#9771) ;
#8856=AXIS2_PLACEMENT_3D('',#112904,#9772,#9773) ;
#8857=AXIS2_PLACEMENT_3D('',#112905,#9774,#9775) ;
#8858=AXIS2_PLACEMENT_3D('',#112907,#9776,#9777) ;
#8859=AXIS2_PLACEMENT_3D('',#112910,#9779,#9780) ;
#8860=AXIS2_PLACEMENT_3D('',#112911,#9781,#9782) ;
#8861=AXIS2_PLACEMENT_3D('',#112913,#9783,#9784) ;
#8862=AXIS2_PLACEMENT_3D('',#112916,#9785,#9786) ;
#8863=AXIS2_PLACEMENT_3D('',#112918,#9787,#9788) ;
#8864=AXIS2_PLACEMENT_3D('',#112920,#9789,#9790) ;
#8865=AXIS2_PLACEMENT_3D('',#112921,#9791,#9792) ;
#8866=AXIS2_PLACEMENT_3D('',#112923,#9793,#9794) ;
#8867=AXIS2_PLACEMENT_3D('',#112926,#9795,#9796) ;
#8868=AXIS2_PLACEMENT_3D('',#112928,#9797,#9798) ;
#8869=AXIS2_PLACEMENT_3D('',#112930,#9799,#9800) ;
#8870=AXIS2_PLACEMENT_3D('',#112931,#9801,#9802) ;
#8871=AXIS2_PLACEMENT_3D('',#112932,#9803,#9804) ;
#8872=AXIS2_PLACEMENT_3D('',#112967,#9805,#9806) ;
#8873=AXIS2_PLACEMENT_3D('',#112980,#9807,#9808) ;
#8874=AXIS2_PLACEMENT_3D('',#112983,#9809,#9810) ;
#8875=AXIS2_PLACEMENT_3D('',#113008,#9811,#9812) ;
#8876=AXIS2_PLACEMENT_3D('',#113038,#9813,#9814) ;
#8877=AXIS2_PLACEMENT_3D('',#113040,#9815,#9816) ;
#8878=AXIS2_PLACEMENT_3D('',#113042,#9818,#9819) ;
#8879=AXIS2_PLACEMENT_3D('',#113058,#9822,#9823) ;
#8880=AXIS2_PLACEMENT_3D('',#113061,#9825,#9826) ;
#8881=AXIS2_PLACEMENT_3D('',#113062,#9827,#9828) ;
#8882=AXIS2_PLACEMENT_3D('',#113076,#9830,#9831) ;
#8883=AXIS2_PLACEMENT_3D('',#113083,#9832,#9833) ;
#8884=AXIS2_PLACEMENT_3D('',#113085,#9834,#9835) ;
#8885=AXIS2_PLACEMENT_3D('',#113087,#9837,#9838) ;
#8886=AXIS2_PLACEMENT_3D('',#113098,#9841,#9842) ;
#8887=AXIS2_PLACEMENT_3D('',#113101,#9844,#9845) ;
#8888=AXIS2_PLACEMENT_3D('',#113102,#9846,#9847) ;
#8889=AXIS2_PLACEMENT_3D('',#113105,#9849,#9850) ;
#8890=AXIS2_PLACEMENT_3D('',#113106,#9851,#9852) ;
#9746=DIRECTION('center_axis',(0.,1.,0.)) ;
#9747=DIRECTION('ref_axis',(0.455018599800652,0.,-0.89048193346943)) ;
#9748=DIRECTION('center_axis',(-2.55214171167663E-16,-1.,4.99460041171382E-16)) ;
#9749=DIRECTION('ref_axis',(0.7484309423753,-5.40804574512742E-16,-0.66321272944299)) ;
#9750=DIRECTION('',(0.,1.,0.)) ;
#9751=DIRECTION('center_axis',(0.,-1.,0.)) ;
#9752=DIRECTION('ref_axis',(0.7484309423753,0.,-0.66321272944299)) ;
#9753=DIRECTION('',(0.,1.,0.)) ;
#9754=DIRECTION('center_axis',(0.,-1.,0.)) ;
#9755=DIRECTION('ref_axis',(0.946102418141935,0.,0.323867587736074)) ;
#9756=DIRECTION('center_axis',(0.,1.,0.)) ;
#9757=DIRECTION('ref_axis',(-0.184992222823419,0.,-0.982739984683055)) ;
#9758=DIRECTION('',(0.,1.,0.)) ;
#9759=DIRECTION('center_axis',(0.,1.,0.)) ;
#9760=DIRECTION('ref_axis',(-0.184992222823419,0.,-0.982739984683055)) ;
#9761=DIRECTION('center_axis',(0.,1.,0.)) ;
#9762=DIRECTION('ref_axis',(-0.186143933560967,0.,0.982522486255887)) ;
#9763=DIRECTION('center_axis',(0.,-1.,0.)) ;
#9764=DIRECTION('ref_axis',(-0.531640234764764,0.,0.846970283291726)) ;
#9765=DIRECTION('',(0.,1.,0.)) ;
#9766=DIRECTION('center_axis',(-1.04405775373722E-16,-1.,5.5108442180881E-16)) ;
#9767=DIRECTION('ref_axis',(-0.531640234764764,5.40804574512721E-16,0.846970283291726)) ;
#9768=DIRECTION('center_axis',(0.,-1.,0.)) ;
#9769=DIRECTION('ref_axis',(-0.946102418141937,0.,-0.323867587736067)) ;
#9770=DIRECTION('center_axis',(0.,1.,0.)) ;
#9771=DIRECTION('ref_axis',(-0.0989310419315636,0.,0.995094291483141)) ;
#9772=DIRECTION('center_axis',(0.,1.,0.)) ;
#9773=DIRECTION('ref_axis',(-0.0989310419315636,0.,0.995094291483141)) ;
#9774=DIRECTION('center_axis',(0.,1.,0.)) ;
#9775=DIRECTION('ref_axis',(-0.99990130540252,0.,0.014049179845692)) ;
#9776=DIRECTION('center_axis',(-8.38487460979998E-16,-1.,-1.63767295998206E-15)) ;
#9777=DIRECTION('ref_axis',(0.80558161685206,0.,-0.592484817181015)) ;
#9778=DIRECTION('',(0.,-1.,0.)) ;
#9779=DIRECTION('center_axis',(-2.99404737873291E-16,-1.,-1.81877242912888E-15)) ;
#9780=DIRECTION('ref_axis',(0.80558161685206,1.11022302462515E-15,-0.592484817181015)) ;
#9781=DIRECTION('center_axis',(0.,-1.,0.)) ;
#9782=DIRECTION('ref_axis',(0.,0.,-1.)) ;
#9783=DIRECTION('center_axis',(2.21922717480124E-16,-1.,-1.77769816013821E-16)) ;
#9784=DIRECTION('ref_axis',(0.552511269382308,0.,-0.833505427220214)) ;
#9785=DIRECTION('center_axis',(-9.60395777197369E-15,-1.,-3.28760405712621E-15)) ;
#9786=DIRECTION('ref_axis',(-0.910070227772796,1.00819783257895E-14,-0.414454075286481)) ;
#9787=DIRECTION('center_axis',(0.,-1.,0.)) ;
#9788=DIRECTION('ref_axis',(-0.973142732923728,0.,-0.230202565923443)) ;
#9789=DIRECTION('center_axis',(-1.22695023382735E-14,1.,-4.20006761299971E-15)) ;
#9790=DIRECTION('ref_axis',(-0.973142645740024,-1.28801978463218E-14,-0.230202934477618)) ;
#9791=DIRECTION('center_axis',(0.,-1.,0.)) ;
#9792=DIRECTION('ref_axis',(0.91007020491951,0.,0.414454125468382)) ;
#9793=DIRECTION('center_axis',(-7.59289697485827E-17,-1.,-2.8895302269988E-17)) ;
#9794=DIRECTION('ref_axis',(0.998564477438101,0.,0.0535629013289298)) ;
#9795=DIRECTION('center_axis',(-1.15689962621907E-15,-1.,-9.23506116525419E-16)) ;
#9796=DIRECTION('ref_axis',(-0.623865270298613,0.,0.781531908827297)) ;
#9797=DIRECTION('center_axis',(-1.66226250514315E-14,1.,1.46874856665111E-14)) ;
#9798=DIRECTION('ref_axis',(-0.62386527029487,-2.17997072578483E-14,0.781531908830284)) ;
#9799=DIRECTION('center_axis',(7.74016996102823E-16,-1.,1.26181600964286E-15)) ;
#9800=DIRECTION('ref_axis',(0.852406595651028,0.,-0.522879523112757)) ;
#9801=DIRECTION('center_axis',(1.14665281872477E-14,-1.,-1.01316426725251E-14)) ;
#9802=DIRECTION('ref_axis',(-0.852406991796352,-1.50377410845894E-14,0.522878877309739)) ;
#9803=DIRECTION('center_axis',(0.,1.,0.)) ;
#9804=DIRECTION('ref_axis',(0.,0.,1.)) ;
#9805=DIRECTION('center_axis',(0.,1.,0.)) ;
#9806=DIRECTION('ref_axis',(-0.323867587734822,0.,0.946102418142364)) ;
#9807=DIRECTION('center_axis',(0.,-1.,0.)) ;
#9808=DIRECTION('ref_axis',(0.323867121549058,0.,-0.946102577725866)) ;
#9809=DIRECTION('center_axis',(0.,-1.,0.)) ;
#9810=DIRECTION('ref_axis',(-0.662139670450416,0.,-0.749380448647957)) ;
#9811=DIRECTION('center_axis',(-3.40221204910911E-14,1.,3.00614012171144E-14)) ;
#9812=DIRECTION('ref_axis',(0.662139806159003,-2.24593216937398E-20,0.749380328738163)) ;
#9813=DIRECTION('center_axis',(0.,1.,0.)) ;
#9814=DIRECTION('ref_axis',(-0.934005212398469,0.,0.357259378060941)) ;
#9815=DIRECTION('center_axis',(0.,-1.,0.)) ;
#9816=DIRECTION('ref_axis',(0.552511269382305,0.,-0.833505427220215)) ;
#9817=DIRECTION('',(0.,-1.,0.)) ;
#9818=DIRECTION('center_axis',(0.,1.,0.)) ;
#9819=DIRECTION('ref_axis',(0.414453894976047,0.,-0.910070309887749)) ;
#9820=DIRECTION('',(0.,1.,0.)) ;
#9821=DIRECTION('',(0.,1.,-6.23283101543947E-15)) ;
#9822=DIRECTION('center_axis',(0.,-1.,0.)) ;
#9823=DIRECTION('ref_axis',(-0.946102418141937,0.,-0.323867587736067)) ;
#9824=DIRECTION('',(0.,1.,6.23283101543947E-15)) ;
#9825=DIRECTION('center_axis',(-2.45390046765453E-14,1.,-8.40013522599877E-15)) ;
#9826=DIRECTION('ref_axis',(-0.973142645740026,-2.58220234335363E-14,-0.23020293447761)) ;
#9827=DIRECTION('center_axis',(0.,1.,0.)) ;
#9828=DIRECTION('ref_axis',(-0.23020275012694,0.,0.973142689349303)) ;
#9829=DIRECTION('',(0.,1.,0.)) ;
#9830=DIRECTION('center_axis',(0.,1.,0.)) ;
#9831=DIRECTION('ref_axis',(-0.946102433711068,0.,-0.323867542254538)) ;
#9832=DIRECTION('center_axis',(0.,1.,0.)) ;
#9833=DIRECTION('ref_axis',(-0.781531908823211,0.,-0.623865270303732)) ;
#9834=DIRECTION('center_axis',(0.,-1.,0.)) ;
#9835=DIRECTION('ref_axis',(0.998564477438101,0.,0.0535629013289298)) ;
#9836=DIRECTION('',(0.,-1.,0.)) ;
#9837=DIRECTION('center_axis',(0.,1.,0.)) ;
#9838=DIRECTION('ref_axis',(-0.749379940776913,0.,0.662140245236)) ;
#9839=DIRECTION('',(0.,1.,0.)) ;
#9840=DIRECTION('',(1.55820775385987E-15,1.,1.2465662030879E-14)) ;
#9841=DIRECTION('center_axis',(0.,1.,0.)) ;
#9842=DIRECTION('ref_axis',(-0.522879200211183,0.,-0.852406793723815)) ;
#9843=DIRECTION('',(0.,1.,0.)) ;
#9844=DIRECTION('center_axis',(-1.40492466406194E-15,-1.,-8.74807498650115E-16)) ;
#9845=DIRECTION('ref_axis',(0.852406595651023,-7.40148683083545E-16,-0.522879523112765)) ;
#9846=DIRECTION('center_axis',(0.,-1.,0.)) ;
#9847=DIRECTION('ref_axis',(-0.749379997167278,0.,0.662140181415967)) ;
#9848=DIRECTION('',(3.11641550771974E-15,1.,0.)) ;
#9849=DIRECTION('center_axis',(1.21477315178064E-14,1.,-1.13769124036181E-14)) ;
#9850=DIRECTION('ref_axis',(-0.623865270294834,1.64745879276906E-14,0.781531908830314)) ;
#9851=DIRECTION('center_axis',(0.,1.,0.)) ;
#9852=DIRECTION('ref_axis',(0.781531908809468,0.,0.623865270320947)) ;
#9853=DIRECTION('',(0.660441423512288,0.70710677669281,-0.252620530567424)) ;
#9854=DIRECTION('',(0.643516813504555,0.707106780936073,0.293063322664521)) ;
#9855=DIRECTION('',(0.643516895788544,-0.707106780933182,0.293063141989894)) ;
#9856=DIRECTION('',(-0.68811576949862,-0.70710677538888,-0.162778057386315)) ;
#9857=DIRECTION('',(-0.688115800926617,0.7071067782106,-0.162777912272352)) ;
#9858=DIRECTION('',(0.552626512834363,0.707106780687659,0.441139363487398)) ;
#9859=DIRECTION('',(-0.602742728927109,0.707106778605105,0.369731262373379)) ;
#9860=DIRECTION('',(0.441139312684097,-0.707106778989338,-0.552626555561643)) ;
#9861=DIRECTION('',(0.602742658952527,0.707106777346419,-0.369731378854432)) ;
#9862=DIRECTION('',(-0.441139363669859,-0.707106780410578,0.552626513043248)) ;
#112881=CARTESIAN_POINT('Origin',(-32.7369214287712,6.20000000004959,159.065417425017)) ;
#112882=CARTESIAN_POINT('',(-29.8935702991225,6.2000000000496,130.4656735525)) ;
#112883=CARTESIAN_POINT('',(-11.2264641357304,6.2000000000496,140.004194424792)) ;
#112884=CARTESIAN_POINT('Origin',(-32.7369214287712,6.20000000004961,159.065417425018)) ;
#112885=CARTESIAN_POINT('',(-11.2264641357304,9.2000000000496,140.004194424792)) ;
#112886=CARTESIAN_POINT('',(-11.2264641357304,6.2000000000496,140.004194424792)) ;
#112887=CARTESIAN_POINT('',(-29.8935702991225,9.2000000000496,130.4656735525)) ;
#112888=CARTESIAN_POINT('Origin',(-32.7369214287712,9.2000000000496,159.065417425018)) ;
#112889=CARTESIAN_POINT('',(-29.8935702991225,6.2000000000496,130.4656735525)) ;
#112890=CARTESIAN_POINT('Origin',(-1.22124532708767E-13,6.2000000000496,
130.056003483261)) ;
#112891=CARTESIAN_POINT('',(-2.77488334235139,6.2000000000496,115.314903713015)) ;
#112892=CARTESIAN_POINT('Origin',(-1.17683640610267E-13,6.2000000000496,
130.056003483261)) ;
#112893=CARTESIAN_POINT('',(-2.77488334235139,9.2000000000496,115.314903713015)) ;
#112894=CARTESIAN_POINT('',(-2.77488334235139,6.2000000000496,115.314903713015)) ;
#112895=CARTESIAN_POINT('Origin',(-1.17683640610267E-13,9.2000000000496,
130.056003483261)) ;
#112896=CARTESIAN_POINT('Origin',(-8.09169626799619,6.2000000000496,87.0702317281284)) ;
#112897=CARTESIAN_POINT('',(-23.3714287291853,6.2000000000496,111.412782357317)) ;
#112898=CARTESIAN_POINT('Origin',(-8.09169626799633,6.2000000000496,87.0702317281289)) ;
#112899=CARTESIAN_POINT('',(-23.3714287291853,9.2000000000496,111.412782357317)) ;
#112900=CARTESIAN_POINT('',(-23.3714287291853,6.2000000000496,111.412782357317)) ;
#112901=CARTESIAN_POINT('Origin',(-8.09169626799633,9.20000000004958,87.0702317281289)) ;
#112902=CARTESIAN_POINT('Origin',(-28.8703041205684,6.2000000000496,120.173187866852)) ;
#112903=CARTESIAN_POINT('Origin',(-28.8703041205685,6.2000000000496,120.173187866852)) ;
#112904=CARTESIAN_POINT('Origin',(-28.8703041205685,9.2000000000496,120.173187866852)) ;
#112905=CARTESIAN_POINT('Origin',(-10.6619859316946,6.2000000000496,134.537724339802)) ;
#112906=CARTESIAN_POINT('',(-9.66208462629207,9.2000000000496,134.523675159956)) ;
#112907=CARTESIAN_POINT('Origin',(-10.6619859316946,9.2000000000496,134.537724339801)) ;
#112908=CARTESIAN_POINT('',(-9.66208462629207,6.2000000000496,134.523675159956)) ;
#112909=CARTESIAN_POINT('',(-9.66208462629206,6.2000000000496,134.523675159956)) ;
#112910=CARTESIAN_POINT('Origin',(-10.6619859316946,6.2000000000496,134.537724339801)) ;
#112911=CARTESIAN_POINT('Origin',(-27.0022936957715,6.2000000000496,119.45866911073)) ;
#112912=CARTESIAN_POINT('',(-27.0022936957715,6.2000000000496,119.45866911073)) ;
#112913=CARTESIAN_POINT('Origin',(-28.8703041205685,6.2000000000496,120.173187866852)) ;
#112914=CARTESIAN_POINT('',(-22.3968667215,6.2000000000496,124.757886585629)) ;
#112915=CARTESIAN_POINT('',(-20.9452555485298,6.2000000000496,120.517347833308)) ;
#112916=CARTESIAN_POINT('Origin',(-4.6047610169353E-11,6.20000000004936,
130.056003483247)) ;
#112917=CARTESIAN_POINT('',(-17.5311532747538,6.2000000000496,125.908900336264)) ;
#112918=CARTESIAN_POINT('Origin',(-19.9640098891908,6.2000000000496,125.333393000437)) ;
#112919=CARTESIAN_POINT('',(-16.3949039990916,6.2000000000496,122.589617308188)) ;
#112920=CARTESIAN_POINT('Origin',(-5.43787237461402E-12,6.20000000004983,
130.056003483259)) ;
#112921=CARTESIAN_POINT('Origin',(-18.6700795113902,6.2000000000496,121.553481994517)) ;
#112922=CARTESIAN_POINT('',(5.47072336176247,6.2000000000496,134.423060375387)) ;
#112923=CARTESIAN_POINT('Origin',(-1.33226762955019E-14,6.2000000000496,
130.056003483261)) ;
#112924=CARTESIAN_POINT('',(-33.0324919366153,6.2000000000496,125.387266520802)) ;
#112925=CARTESIAN_POINT('',(-34.9040877475781,6.2000000000496,127.731862247231)) ;
#112926=CARTESIAN_POINT('Origin',(-33.9682898421302,6.2000000000496,126.55956438399)) ;
#112927=CARTESIAN_POINT('',(-34.557234512772,6.2000000000496,123.661632554657)) ;
#112928=CARTESIAN_POINT('Origin',(-28.8703041205576,6.20000000004974,120.173187866839)) ;
#112929=CARTESIAN_POINT('',(-37.1144548939429,6.2000000000496,125.23027015529)) ;
#112930=CARTESIAN_POINT('Origin',(-35.8358444062484,6.2000000000496,124.445951839326)) ;
#112931=CARTESIAN_POINT('Origin',(-28.8703041205676,6.20000000004974,120.173187866851)) ;
#112932=CARTESIAN_POINT('Origin',(-27.0022936957715,9.2000000000496,119.45866911073)) ;
#112933=CARTESIAN_POINT('',(5.58795314825178,9.2000000000496,134.516640166064)) ;
#112934=CARTESIAN_POINT('Ctrl Pts',(5.58795314825178,9.2000000000496,134.516640166064)) ;
#112935=CARTESIAN_POINT('Ctrl Pts',(5.02776600408638,9.2000000000496,135.218925186777)) ;
#112936=CARTESIAN_POINT('Ctrl Pts',(3.58102682874936,9.20000000004958,136.459065126737)) ;
#112937=CARTESIAN_POINT('Ctrl Pts',(0.819706526786835,9.2000000000496,137.362239934218)) ;
#112938=CARTESIAN_POINT('Ctrl Pts',(-2.07329727026273,9.20000000004959,
137.093448346514)) ;
#112939=CARTESIAN_POINT('Ctrl Pts',(-4.56753011885253,9.20000000004959,
135.777900274175)) ;
#112940=CARTESIAN_POINT('Ctrl Pts',(-6.40313455515177,9.2000000000496,133.637111179546)) ;
#112941=CARTESIAN_POINT('Ctrl Pts',(-7.30617826165478,9.20000000004959,
130.875683925058)) ;
#112942=CARTESIAN_POINT('Ctrl Pts',(-7.03751608684004,9.20000000004958,
127.982693648484)) ;
#112943=CARTESIAN_POINT('Ctrl Pts',(-5.72184342923753,9.2000000000496,125.488474550351)) ;
#112944=CARTESIAN_POINT('Ctrl Pts',(-3.5811627186061,9.20000000004957,123.652885698944)) ;
#112945=CARTESIAN_POINT('Ctrl Pts',(-0.819600541308432,9.2000000000496,
122.749780638574)) ;
#112946=CARTESIAN_POINT('Ctrl Pts',(2.07323217291338,9.20000000004958,123.018548271325)) ;
#112947=CARTESIAN_POINT('Ctrl Pts',(4.56757555136914,9.20000000004958,124.334122518572)) ;
#112948=CARTESIAN_POINT('Ctrl Pts',(6.4030863521721,9.20000000004959,126.474865718472)) ;
#112949=CARTESIAN_POINT('Ctrl Pts',(7.30625034559879,9.20000000004959,129.236381983343)) ;
#112950=CARTESIAN_POINT('Ctrl Pts',(7.03738575174059,9.2000000000496,132.129195828704)) ;
#112951=CARTESIAN_POINT('Ctrl Pts',(6.14865293878678,9.20000000004959,133.814761812278)) ;
#112952=CARTESIAN_POINT('Ctrl Pts',(5.58795314825178,9.2000000000496,134.516640166064)) ;
#112953=CARTESIAN_POINT('',(-21.0817660968248,9.2000000000496,120.455179752781)) ;
#112954=CARTESIAN_POINT('',(-16.2583934682522,9.2000000000496,122.651785427042)) ;
#112955=CARTESIAN_POINT('Ctrl Pts',(-21.0817660968248,9.2000000000496,120.455179752781)) ;
#112956=CARTESIAN_POINT('Ctrl Pts',(-20.9381930117988,9.2000000000496,120.13944913774)) ;
#112957=CARTESIAN_POINT('Ctrl Pts',(-20.5249581888851,9.2000000000496,119.56540103953)) ;
#112958=CARTESIAN_POINT('Ctrl Pts',(-19.6230264687625,9.20000000004958,
119.006828830265)) ;
#112959=CARTESIAN_POINT('Ctrl Pts',(-18.5758907605794,9.2000000000496,118.83604139381)) ;
#112960=CARTESIAN_POINT('Ctrl Pts',(-17.5431612788873,9.20000000004959,
119.078919711506)) ;
#112961=CARTESIAN_POINT('Ctrl Pts',(-16.6819548364584,9.20000000004959,
119.698549065317)) ;
#112962=CARTESIAN_POINT('Ctrl Pts',(-16.123420065397,9.2000000000496,120.60057414181)) ;
#112963=CARTESIAN_POINT('Ctrl Pts',(-15.9526858401603,9.20000000004958,
121.647648458748)) ;
#112964=CARTESIAN_POINT('Ctrl Pts',(-16.1144562107074,9.2000000000496,122.336195813076)) ;
#112965=CARTESIAN_POINT('Ctrl Pts',(-16.2583934681596,9.2000000000496,122.651785427097)) ;
#112966=CARTESIAN_POINT('',(-17.3851818756338,9.19999999991291,125.943430776977)) ;
#112967=CARTESIAN_POINT('Origin',(-4.21641852046444,9.2000000000496,128.61264886444)) ;
#112968=CARTESIAN_POINT('',(-22.5428381268374,9.2000000000496,124.723356175805)) ;
#112969=CARTESIAN_POINT('Ctrl Pts',(-17.3851818731081,9.2000000000496,125.943430777582)) ;
#112970=CARTESIAN_POINT('Ctrl Pts',(-17.4648341623564,9.20000000004959,
126.281003578961)) ;
#112971=CARTESIAN_POINT('Ctrl Pts',(-17.7589736989414,9.20000000004959,
126.924250687851)) ;
#112972=CARTESIAN_POINT('Ctrl Pts',(-18.5355338243201,9.2000000000496,127.647054501784)) ;
#112973=CARTESIAN_POINT('Ctrl Pts',(-19.5297170934661,9.2000000000496,128.017558118363)) ;
#112974=CARTESIAN_POINT('Ctrl Pts',(-20.5899333565814,9.2000000000496,127.979449233406)) ;
#112975=CARTESIAN_POINT('Ctrl Pts',(-21.5549025420905,9.2000000000496,127.538495083066)) ;
#112976=CARTESIAN_POINT('Ctrl Pts',(-22.2776843192047,9.2000000000496,126.761830817273)) ;
#112977=CARTESIAN_POINT('Ctrl Pts',(-22.6481211896443,9.20000000004961,
125.767700230883)) ;
#112978=CARTESIAN_POINT('Ctrl Pts',(-22.6228797294498,9.2000000000496,125.06085865435)) ;
#112979=CARTESIAN_POINT('Ctrl Pts',(-22.5428381268374,9.2000000000496,124.723356175805)) ;
#112980=CARTESIAN_POINT('Origin',(-5.46730784800664,9.2000000000496,128.184450336603)) ;
#112981=CARTESIAN_POINT('',(-34.9976674182864,9.2000000000496,127.849092131696)) ;
#112982=CARTESIAN_POINT('',(-37.2423156796051,9.2000000000496,125.308702418377)) ;
#112983=CARTESIAN_POINT('Origin',(-30.6977563686737,9.2000000000496,121.787893254627)) ;
#112984=CARTESIAN_POINT('',(-34.4293734856409,9.2000000000496,123.583200684669)) ;
#112985=CARTESIAN_POINT('Ctrl Pts',(-37.2423156796052,9.2000000000496,125.308702418377)) ;
#112986=CARTESIAN_POINT('Ctrl Pts',(-37.3035108477935,9.2000000000496,125.210394441041)) ;
#112987=CARTESIAN_POINT('Ctrl Pts',(-37.3534324664497,9.20000000004957,
125.1053745779)) ;
#112988=CARTESIAN_POINT('Ctrl Pts',(-37.4300532165178,9.20000000004957,
124.886985389158)) ;
#112989=CARTESIAN_POINT('Ctrl Pts',(-37.4567166242111,9.20000000004957,
124.773812893931)) ;
#112990=CARTESIAN_POINT('Ctrl Pts',(-37.4967079950417,9.20000000004957,
124.464620592181)) ;
#112991=CARTESIAN_POINT('Ctrl Pts',(-37.489671697536,9.20000000004957,124.252609113297)) ;
#112992=CARTESIAN_POINT('Ctrl Pts',(-37.3824674523358,9.20000000004957,
123.831470024454)) ;
#112993=CARTESIAN_POINT('Ctrl Pts',(-37.2886173018908,9.20000000004956,
123.634993007773)) ;
#112994=CARTESIAN_POINT('Ctrl Pts',(-37.035690031635,9.20000000004956,123.294197445114)) ;
#112995=CARTESIAN_POINT('Ctrl Pts',(-36.8780104418293,9.20000000004958,
123.149398131845)) ;
#112996=CARTESIAN_POINT('Ctrl Pts',(-36.5193687649608,9.20000000004958,
122.929404397955)) ;
#112997=CARTESIAN_POINT('Ctrl Pts',(-36.3186607801125,9.20000000004958,
122.854370983339)) ;
#112998=CARTESIAN_POINT('Ctrl Pts',(-35.9005416749946,9.20000000004958,
122.78339315007)) ;
#112999=CARTESIAN_POINT('Ctrl Pts',(-35.6833683383588,9.20000000004958,
122.788791264233)) ;
#113000=CARTESIAN_POINT('Ctrl Pts',(-35.2593825552086,9.20000000004958,
122.883888816214)) ;
#113001=CARTESIAN_POINT('Ctrl Pts',(-35.0667355944975,9.20000000004958,
122.973751721585)) ;
#113002=CARTESIAN_POINT('Ctrl Pts',(-34.8088104674519,9.20000000004958,
123.149773346661)) ;
#113003=CARTESIAN_POINT('Ctrl Pts',(-34.7200310044914,9.20000000004958,
123.224791694348)) ;
#113004=CARTESIAN_POINT('Ctrl Pts',(-34.5601404915692,9.20000000004958,
123.392015869226)) ;
#113005=CARTESIAN_POINT('Ctrl Pts',(-34.4891960629546,9.2000000000496,123.484094170402)) ;
#113006=CARTESIAN_POINT('Ctrl Pts',(-34.4293734856409,9.2000000000496,123.583200684669)) ;
#113007=CARTESIAN_POINT('',(-32.9389121458628,9.2000000000496,125.270036734223)) ;
#113008=CARTESIAN_POINT('Origin',(-30.0837635005368,9.20000000004981,121.24538010296)) ;
#113009=CARTESIAN_POINT('Ctrl Pts',(-32.9389121456355,9.2000000000496,125.270036733944)) ;
#113010=CARTESIAN_POINT('Ctrl Pts',(-32.5987066128391,9.2000000000496,125.537972355178)) ;
#113011=CARTESIAN_POINT('Ctrl Pts',(-32.2656287248248,9.2000000000496,126.150548345613)) ;
#113012=CARTESIAN_POINT('Ctrl Pts',(-32.3422999176508,9.2000000000496,127.029372379786)) ;
#113013=CARTESIAN_POINT('Ctrl Pts',(-32.6448691671967,9.2000000000496,127.615804974768)) ;
#113014=CARTESIAN_POINT('Ctrl Pts',(-33.1500786747586,9.2000000000496,128.041286812588)) ;
#113015=CARTESIAN_POINT('Ctrl Pts',(-33.9896462617629,9.2000000000496,128.310218608482)) ;
#113016=CARTESIAN_POINT('Ctrl Pts',(-34.6611211806255,9.20000000004961,
128.121705182437)) ;
#113017=CARTESIAN_POINT('Ctrl Pts',(-34.9976674182864,9.2000000000496,127.849092131696)) ;
#113018=CARTESIAN_POINT('',(-26.8621929121386,9.2000000000496,119.40508020332)) ;
#113019=CARTESIAN_POINT('Ctrl Pts',(-26.8621929121386,9.2000000000496,119.40508020332)) ;
#113020=CARTESIAN_POINT('Ctrl Pts',(-26.7615104285989,9.20000000004959,
119.667852759595)) ;
#113021=CARTESIAN_POINT('Ctrl Pts',(-26.6651414372152,9.2000000000496,120.233557031884)) ;
#113022=CARTESIAN_POINT('Ctrl Pts',(-26.8560141325428,9.2000000000496,121.072849900875)) ;
#113023=CARTESIAN_POINT('Ctrl Pts',(-27.3536755345133,9.2000000000496,121.775201700263)) ;
#113024=CARTESIAN_POINT('Ctrl Pts',(-28.0821610405967,9.2000000000496,122.233641256589)) ;
#113025=CARTESIAN_POINT('Ctrl Pts',(-28.9306655937973,9.20000000004959,
122.378411352712)) ;
#113026=CARTESIAN_POINT('Ctrl Pts',(-29.769968345177,9.20000000004959,122.187446863389)) ;
#113027=CARTESIAN_POINT('Ctrl Pts',(-30.4723169970674,9.20000000004959,
121.689833204347)) ;
#113028=CARTESIAN_POINT('Ctrl Pts',(-30.9307580101565,9.20000000004961,
120.961321719305)) ;
#113029=CARTESIAN_POINT('Ctrl Pts',(-31.0755273221357,9.20000000004959,
120.112831708247)) ;
#113030=CARTESIAN_POINT('Ctrl Pts',(-30.8845632771364,9.20000000004961,
119.27352063753)) ;
#113031=CARTESIAN_POINT('Ctrl Pts',(-30.3869493696082,9.20000000004959,
118.571176652922)) ;
#113032=CARTESIAN_POINT('Ctrl Pts',(-29.6584380217711,9.20000000004961,
118.112733056803)) ;
#113033=CARTESIAN_POINT('Ctrl Pts',(-28.8099464114727,9.2000000000496,117.967965846063)) ;
#113034=CARTESIAN_POINT('Ctrl Pts',(-27.9706124163009,9.20000000004959,
118.15891731463)) ;
#113035=CARTESIAN_POINT('Ctrl Pts',(-27.2683350105885,9.2000000000496,118.656574828484)) ;
#113036=CARTESIAN_POINT('Ctrl Pts',(-26.9625809346018,9.2000000000496,119.142176892536)) ;
#113037=CARTESIAN_POINT('Ctrl Pts',(-26.8621929121386,9.2000000000496,119.40508020332)) ;
#113038=CARTESIAN_POINT('Origin',(-28.8703041205685,6.2000000000496,120.173187866852)) ;
#113039=CARTESIAN_POINT('',(-27.0022936957715,9.05000000004959,119.45866911073)) ;
#113040=CARTESIAN_POINT('Origin',(-28.8703041205685,9.05000000004959,120.173187866852)) ;
#113041=CARTESIAN_POINT('',(-27.0022936957716,6.2000000000496,119.45866911073)) ;
#113042=CARTESIAN_POINT('Origin',(-18.6700795113902,6.2000000000496,121.553481994517)) ;
#113043=CARTESIAN_POINT('',(-20.9452555485298,9.05000000004959,120.517347833308)) ;
#113044=CARTESIAN_POINT('',(-20.9452555485298,6.2000000000496,120.517347833308)) ;
#113045=CARTESIAN_POINT('',(-16.3949039990916,9.05000000004959,122.589617308188)) ;
#113046=CARTESIAN_POINT('',(-16.3949039990916,6.2000000000496,122.589617308188)) ;
#113047=CARTESIAN_POINT('Ctrl Pts',(-20.9452555485298,9.05000000004959,
120.517347833308)) ;
#113048=CARTESIAN_POINT('Ctrl Pts',(-20.8098092259609,9.05000000004959,
120.219488731387)) ;
#113049=CARTESIAN_POINT('Ctrl Pts',(-20.4199650586345,9.0500000000496,119.677933924817)) ;
#113050=CARTESIAN_POINT('Ctrl Pts',(-19.5690860737905,9.05000000004958,
119.150979010872)) ;
#113051=CARTESIAN_POINT('Ctrl Pts',(-18.5812221993204,9.05000000004961,
118.989858785028)) ;
#113052=CARTESIAN_POINT('Ctrl Pts',(-17.606949105008,9.05000000004959,119.218989276765)) ;
#113053=CARTESIAN_POINT('Ctrl Pts',(-16.7944901933067,9.05000000004959,
119.803545268697)) ;
#113054=CARTESIAN_POINT('Ctrl Pts',(-16.2675706030868,9.05000000004959,
120.65451232145)) ;
#113055=CARTESIAN_POINT('Ctrl Pts',(-16.1065005744166,9.05000000004958,
121.642318285021)) ;
#113056=CARTESIAN_POINT('Ctrl Pts',(-16.2591141342633,9.0500000000496,122.291891253157)) ;
#113057=CARTESIAN_POINT('Ctrl Pts',(-16.3949039990916,9.05000000004959,
122.589617308188)) ;
#113058=CARTESIAN_POINT('Origin',(-4.34985381048136E-12,6.20000000004959,
130.056003483259)) ;
#113059=CARTESIAN_POINT('',(-17.5311532747538,9.05000000004959,125.908900336264)) ;
#113060=CARTESIAN_POINT('',(-17.5311532747538,6.2000000000496,125.908900336264)) ;
#113061=CARTESIAN_POINT('Origin',(-6.26387830493513E-12,9.05000000005006,
130.056003483259)) ;
#113062=CARTESIAN_POINT('Origin',(-19.9640098891908,6.2000000000496,125.333393000437)) ;
#113063=CARTESIAN_POINT('',(-22.3968667215,9.05000000004959,124.757886585629)) ;
#113064=CARTESIAN_POINT('',(-22.3968667215,6.2000000000496,124.757886585629)) ;
#113065=CARTESIAN_POINT('Ctrl Pts',(-17.5311532747538,9.05000000004959,
125.908900336264)) ;
#113066=CARTESIAN_POINT('Ctrl Pts',(-17.6062969361899,9.05000000004959,
126.227365244915)) ;
#113067=CARTESIAN_POINT('Ctrl Pts',(-17.8837870704631,9.05000000004959,
126.834202139267)) ;
#113068=CARTESIAN_POINT('Ctrl Pts',(-18.6163909589713,9.05000000004961,
127.516092529978)) ;
#113069=CARTESIAN_POINT('Ctrl Pts',(-19.5542997048764,9.0500000000496,127.865624243821)) ;
#113070=CARTESIAN_POINT('Ctrl Pts',(-20.5545037267052,9.0500000000496,127.829672465207)) ;
#113071=CARTESIAN_POINT('Ctrl Pts',(-21.4648520142714,9.0500000000496,127.413677984308)) ;
#113072=CARTESIAN_POINT('Ctrl Pts',(-22.1467216161347,9.05000000004959,
126.680975846054)) ;
#113073=CARTESIAN_POINT('Ctrl Pts',(-22.4961903603291,9.05000000004961,
125.743116803329)) ;
#113074=CARTESIAN_POINT('Ctrl Pts',(-22.4723776645545,9.05000000004959,
125.076285126214)) ;
#113075=CARTESIAN_POINT('Ctrl Pts',(-22.3968667215,9.05000000004959,124.757886585629)) ;
#113076=CARTESIAN_POINT('Origin',(-4.80682160741708E-11,6.2000000000496,
130.056003483246)) ;
#113077=CARTESIAN_POINT('Ctrl Pts',(-22.3968667215,9.05000000004959,124.757886585629)) ;
#113078=CARTESIAN_POINT('Ctrl Pts',(-22.2245939589431,9.049950612143,124.029633476594)) ;
#113079=CARTESIAN_POINT('Ctrl Pts',(-22.0169038912293,9.05001239481549,
123.310215297127)) ;
#113080=CARTESIAN_POINT('Ctrl Pts',(-21.5321687944225,9.05001239481544,
121.894176346136)) ;
#113081=CARTESIAN_POINT('Ctrl Pts',(-21.2554130236569,9.04995061214263,
121.198400574409)) ;
#113082=CARTESIAN_POINT('Ctrl Pts',(-20.9452555485298,9.05000000004959,
120.517347833308)) ;
#113083=CARTESIAN_POINT('Origin',(-4.21884749357559E-14,6.2000000000496,
130.056003483261)) ;
#113084=CARTESIAN_POINT('',(5.47072336176247,9.05000000004959,134.423060375387)) ;
#113085=CARTESIAN_POINT('Origin',(-1.4432899320127E-14,9.05000000004959,
130.056003483261)) ;
#113086=CARTESIAN_POINT('',(5.47072336176241,6.2000000000496,134.423060375387)) ;
#113087=CARTESIAN_POINT('Origin',(-28.8703041205676,6.20000000004959,120.173187866851)) ;
#113088=CARTESIAN_POINT('',(-34.9040876899405,9.04999999949199,127.731862293537)) ;
#113089=CARTESIAN_POINT('',(-34.9040877475781,6.2000000000496,127.731862247231)) ;
#113090=CARTESIAN_POINT('',(-37.1144547230141,9.04999999990636,125.230270433971)) ;
#113091=CARTESIAN_POINT('',(-37.1144548939429,6.2000000000496,125.23027015529)) ;
#113092=CARTESIAN_POINT('Ctrl Pts',(-34.9040876897959,9.04999999901832,
127.731862293356)) ;
#113093=CARTESIAN_POINT('Ctrl Pts',(-35.3413645465505,9.04979412705185,
127.382801894057)) ;
#113094=CARTESIAN_POINT('Ctrl Pts',(-35.7475313924077,9.05005211409003,
126.996450959224)) ;
#113095=CARTESIAN_POINT('Ctrl Pts',(-36.4885024120155,9.05005211928734,
126.157853987428)) ;
#113096=CARTESIAN_POINT('Ctrl Pts',(-36.8218973505677,9.04979413761622,
125.707202917238)) ;
#113097=CARTESIAN_POINT('Ctrl Pts',(-37.1144546376467,9.0499999998019,125.230270573109)) ;
#113098=CARTESIAN_POINT('Origin',(-35.8358444062483,6.2000000000496,124.445951839326)) ;
#113099=CARTESIAN_POINT('',(-34.557234512772,9.05000000004959,123.661632554657)) ;
#113100=CARTESIAN_POINT('',(-34.557234512772,6.2000000000496,123.661632554657)) ;
#113101=CARTESIAN_POINT('Origin',(-35.8358444062484,9.05000000004959,124.445951839326)) ;
#113102=CARTESIAN_POINT('Origin',(-28.8703041205587,6.20000000004959,120.17318786684)) ;
#113103=CARTESIAN_POINT('',(-33.0324919366153,9.05000000004959,125.387266520802)) ;
#113104=CARTESIAN_POINT('',(-33.0324919366153,6.2000000000496,125.387266520802)) ;
#113105=CARTESIAN_POINT('Origin',(-28.8703041205587,9.05000000004948,120.17318786684)) ;
#113106=CARTESIAN_POINT('Origin',(-33.9682898421302,6.2000000000496,126.55956438399)) ;
#113107=CARTESIAN_POINT('Ctrl Pts',(-33.0324919366153,9.05000000004959,
125.387266520802)) ;
#113108=CARTESIAN_POINT('Ctrl Pts',(-32.7232141786532,9.05000000004961,
125.630844357595)) ;
#113109=CARTESIAN_POINT('Ctrl Pts',(-32.4204161032166,9.05000000004959,
126.187731618834)) ;
#113110=CARTESIAN_POINT('Ctrl Pts',(-32.4901171977394,9.0500000000496,126.986662550358)) ;
#113111=CARTESIAN_POINT('Ctrl Pts',(-32.7651801608489,9.0500000000496,127.519783083619)) ;
#113112=CARTESIAN_POINT('Ctrl Pts',(-33.2244615410704,9.0500000000496,127.906584747446)) ;
#113113=CARTESIAN_POINT('Ctrl Pts',(-33.98770481185,9.0500000000496,128.151068188889)) ;
#113114=CARTESIAN_POINT('Ctrl Pts',(-34.5981365609726,9.0500000000496,127.979692345601)) ;
#113115=CARTESIAN_POINT('Ctrl Pts',(-34.9040876850543,9.05000000004959,
127.731862297877)) ;
#113116=CARTESIAN_POINT('Ctrl Pts',(-27.0096412809262,9.04213325052386,
119.46147958081)) ;
#113117=CARTESIAN_POINT('Ctrl Pts',(-26.8621929121386,9.2000000000496,119.40508020332)) ;
#113118=CARTESIAN_POINT('Ctrl Pts',(-26.9163515465784,9.04213325052386,
119.704957694364)) ;
#113119=CARTESIAN_POINT('Ctrl Pts',(-26.7615104285989,9.20000000004959,
119.667852759595)) ;
#113120=CARTESIAN_POINT('Ctrl Pts',(-26.8270585844507,9.04213325052387,
120.22912434222)) ;
#113121=CARTESIAN_POINT('Ctrl Pts',(-26.6651414372152,9.2000000000496,120.233557031884)) ;
#113122=CARTESIAN_POINT('Ctrl Pts',(-27.0039161850776,9.04213325052386,
121.006790961142)) ;
#113123=CARTESIAN_POINT('Ctrl Pts',(-26.8560141325428,9.2000000000496,121.072849900875)) ;
#113124=CARTESIAN_POINT('Ctrl Pts',(-27.4650361038947,9.04213325052387,
121.657571599361)) ;
#113125=CARTESIAN_POINT('Ctrl Pts',(-27.3536755345133,9.2000000000496,121.775201700263)) ;
#113126=CARTESIAN_POINT('Ctrl Pts',(-28.1400315464981,9.04213325052387,
122.082349592043)) ;
#113127=CARTESIAN_POINT('Ctrl Pts',(-28.0821610405967,9.2000000000496,122.233641256589)) ;
#113128=CARTESIAN_POINT('Ctrl Pts',(-28.9262334681465,9.04213325052386,
122.216489741491)) ;
#113129=CARTESIAN_POINT('Ctrl Pts',(-28.9306655937973,9.20000000004959,
122.378411352712)) ;
#113130=CARTESIAN_POINT('Ctrl Pts',(-29.7039092450077,9.04213325052386,
122.03954708619)) ;
#113131=CARTESIAN_POINT('Ctrl Pts',(-29.769968345177,9.20000000004959,122.187446863389)) ;
#113132=CARTESIAN_POINT('Ctrl Pts',(-30.3546869661086,9.04213325052386,
121.578471404859)) ;
#113133=CARTESIAN_POINT('Ctrl Pts',(-30.4723169970674,9.20000000004959,
121.689833204347)) ;
#113134=CARTESIAN_POINT('Ctrl Pts',(-30.7794663090683,9.04213325052388,
120.903451890977)) ;
#113135=CARTESIAN_POINT('Ctrl Pts',(-30.9307580101565,9.20000000004961,
120.961321719305)) ;
#113136=CARTESIAN_POINT('Ctrl Pts',(-30.9136057317632,9.04213325052386,
120.117263443625)) ;
#113137=CARTESIAN_POINT('Ctrl Pts',(-31.0755273221357,9.20000000004959,
120.112831708247)) ;
#113138=CARTESIAN_POINT('Ctrl Pts',(-30.7366634886015,9.04213325052388,
119.33957995907)) ;
#113139=CARTESIAN_POINT('Ctrl Pts',(-30.8845632771364,9.20000000004961,
119.27352063753)) ;
#113140=CARTESIAN_POINT('Ctrl Pts',(-30.2755875763735,9.04213325052386,
118.688806561695)) ;
#113141=CARTESIAN_POINT('Ctrl Pts',(-30.3869493696082,9.20000000004959,
118.571176652922)) ;
#113142=CARTESIAN_POINT('Ctrl Pts',(-29.6005681904104,9.04213325052388,
118.264024825605)) ;
#113143=CARTESIAN_POINT('Ctrl Pts',(-29.6584380217711,9.20000000004961,
118.112733056803)) ;
#113144=CARTESIAN_POINT('Ctrl Pts',(-28.8143782605279,9.04213325052386,
118.129887349728)) ;
#113145=CARTESIAN_POINT('Ctrl Pts',(-28.8099464114727,9.2000000000496,117.967965846063)) ;
#113146=CARTESIAN_POINT('Ctrl Pts',(-28.0366735347411,9.04213325052387,
118.306817939836)) ;
#113147=CARTESIAN_POINT('Ctrl Pts',(-27.9706124163009,9.20000000004959,
118.15891731463)) ;
#113148=CARTESIAN_POINT('Ctrl Pts',(-27.385961828654,9.04213325052387,118.7679342568)) ;
#113149=CARTESIAN_POINT('Ctrl Pts',(-27.2683350105885,9.2000000000496,118.656574828484)) ;
#113150=CARTESIAN_POINT('Ctrl Pts',(-27.1026581693672,9.04213325052387,
119.217880311326)) ;
#113151=CARTESIAN_POINT('Ctrl Pts',(-26.9625809346018,9.2000000000496,119.142176892536)) ;
#113152=CARTESIAN_POINT('Ctrl Pts',(-27.0096412809262,9.04213325052386,
119.46147958081)) ;
#113153=CARTESIAN_POINT('Ctrl Pts',(-26.8621929121386,9.2000000000496,119.40508020332)) ;
#113154=CARTESIAN_POINT('',(-27.0022936957715,9.05000000004959,119.45866911073)) ;
#113155=CARTESIAN_POINT('Ctrl Pts',(-20.9452555485298,9.05000000004959,
120.517347833308)) ;
#113156=CARTESIAN_POINT('Ctrl Pts',(-21.0817660968248,9.2000000000496,120.455179752781)) ;
#113157=CARTESIAN_POINT('Ctrl Pts',(-20.8098092259609,9.05000000004959,
120.219488731387)) ;
#113158=CARTESIAN_POINT('Ctrl Pts',(-20.9381930117988,9.2000000000496,120.13944913774)) ;
#113159=CARTESIAN_POINT('Ctrl Pts',(-20.4199650586345,9.0500000000496,119.677933924817)) ;
#113160=CARTESIAN_POINT('Ctrl Pts',(-20.5249581888851,9.2000000000496,119.56540103953)) ;
#113161=CARTESIAN_POINT('Ctrl Pts',(-19.5690860737905,9.05000000004958,
119.150979010872)) ;
#113162=CARTESIAN_POINT('Ctrl Pts',(-19.6230264687625,9.20000000004958,
119.006828830265)) ;
#113163=CARTESIAN_POINT('Ctrl Pts',(-18.5812221993204,9.05000000004961,
118.989858785028)) ;
#113164=CARTESIAN_POINT('Ctrl Pts',(-18.5758907605794,9.2000000000496,118.83604139381)) ;
#113165=CARTESIAN_POINT('Ctrl Pts',(-17.606949105008,9.05000000004959,119.218989276765)) ;
#113166=CARTESIAN_POINT('Ctrl Pts',(-17.5431612788873,9.20000000004959,
119.078919711506)) ;
#113167=CARTESIAN_POINT('Ctrl Pts',(-16.7944901933067,9.05000000004959,
119.803545268697)) ;
#113168=CARTESIAN_POINT('Ctrl Pts',(-16.6819548364584,9.20000000004959,
119.698549065317)) ;
#113169=CARTESIAN_POINT('Ctrl Pts',(-16.2675706030868,9.05000000004959,
120.65451232145)) ;
#113170=CARTESIAN_POINT('Ctrl Pts',(-16.123420065397,9.2000000000496,120.60057414181)) ;
#113171=CARTESIAN_POINT('Ctrl Pts',(-16.1065005744166,9.05000000004958,
121.642318285021)) ;
#113172=CARTESIAN_POINT('Ctrl Pts',(-15.9526858401603,9.20000000004958,
121.647648458748)) ;
#113173=CARTESIAN_POINT('Ctrl Pts',(-16.2591141342633,9.0500000000496,122.291891253157)) ;
#113174=CARTESIAN_POINT('Ctrl Pts',(-16.1144562107074,9.2000000000496,122.336195813076)) ;
#113175=CARTESIAN_POINT('Ctrl Pts',(-16.3949039990916,9.05000000004959,
122.589617308188)) ;
#113176=CARTESIAN_POINT('Ctrl Pts',(-16.2583934681596,9.2000000000496,122.651785427097)) ;
#113177=CARTESIAN_POINT('',(-16.3949039990916,9.05000000004959,122.589617308188)) ;
#113178=CARTESIAN_POINT('',(-21.0817660968248,9.2000000000496,120.455179752781)) ;
#113179=CARTESIAN_POINT('Ctrl Pts',(-16.3949039990916,9.05000000004959,
122.589617308188)) ;
#113180=CARTESIAN_POINT('Ctrl Pts',(-16.2583934683448,9.2000000000496,122.651785426988)) ;
#113181=CARTESIAN_POINT('Ctrl Pts',(-16.8804331897068,9.0500000000496,123.655569656133)) ;
#113182=CARTESIAN_POINT('Ctrl Pts',(-16.7398799486352,9.20000000004959,
123.708862229139)) ;
#113183=CARTESIAN_POINT('Ctrl Pts',(-17.2615869582204,9.05000000004959,
124.769020077632)) ;
#113184=CARTESIAN_POINT('Ctrl Pts',(-17.1178600783809,9.2000000000496,124.813041616962)) ;
#113185=CARTESIAN_POINT('Ctrl Pts',(-17.5311532747538,9.05000000004959,
125.908900336264)) ;
#113186=CARTESIAN_POINT('Ctrl Pts',(-17.3851818778934,9.2000000000496,125.943430776435)) ;
#113187=CARTESIAN_POINT('',(-17.3851818755008,9.2000000000496,125.943430777009)) ;
#113188=CARTESIAN_POINT('Ctrl Pts',(-17.5311532747538,9.05000000004959,
125.908900336264)) ;
#113189=CARTESIAN_POINT('Ctrl Pts',(-17.3851818731081,9.2000000000496,125.943430777582)) ;
#113190=CARTESIAN_POINT('Ctrl Pts',(-17.6062969361899,9.05000000004959,
126.227365244915)) ;
#113191=CARTESIAN_POINT('Ctrl Pts',(-17.4648341623564,9.20000000004959,
126.281003578961)) ;
#113192=CARTESIAN_POINT('Ctrl Pts',(-17.8837870704631,9.05000000004959,
126.834202139267)) ;
#113193=CARTESIAN_POINT('Ctrl Pts',(-17.7589736989414,9.20000000004959,
126.924250687851)) ;
#113194=CARTESIAN_POINT('Ctrl Pts',(-18.6163909589713,9.05000000004961,
127.516092529978)) ;
#113195=CARTESIAN_POINT('Ctrl Pts',(-18.5355338243201,9.2000000000496,127.647054501784)) ;
#113196=CARTESIAN_POINT('Ctrl Pts',(-19.5542997048764,9.0500000000496,127.865624243821)) ;
#113197=CARTESIAN_POINT('Ctrl Pts',(-19.5297170934661,9.2000000000496,128.017558118363)) ;
#113198=CARTESIAN_POINT('Ctrl Pts',(-20.5545037267052,9.0500000000496,127.829672465207)) ;
#113199=CARTESIAN_POINT('Ctrl Pts',(-20.5899333565814,9.2000000000496,127.979449233406)) ;
#113200=CARTESIAN_POINT('Ctrl Pts',(-21.4648520142714,9.0500000000496,127.413677984308)) ;
#113201=CARTESIAN_POINT('Ctrl Pts',(-21.5549025420905,9.2000000000496,127.538495083066)) ;
#113202=CARTESIAN_POINT('Ctrl Pts',(-22.1467216161347,9.05000000004959,
126.680975846054)) ;
#113203=CARTESIAN_POINT('Ctrl Pts',(-22.2776843192047,9.2000000000496,126.761830817273)) ;
#113204=CARTESIAN_POINT('Ctrl Pts',(-22.4961903603291,9.05000000004961,
125.743116803329)) ;
#113205=CARTESIAN_POINT('Ctrl Pts',(-22.6481211896443,9.20000000004961,
125.767700230883)) ;
#113206=CARTESIAN_POINT('Ctrl Pts',(-22.4723776645545,9.05000000004959,
125.076285126214)) ;
#113207=CARTESIAN_POINT('Ctrl Pts',(-22.6228797294498,9.2000000000496,125.06085865435)) ;
#113208=CARTESIAN_POINT('Ctrl Pts',(-22.3968667215,9.05000000004959,124.757886585629)) ;
#113209=CARTESIAN_POINT('Ctrl Pts',(-22.5428381268374,9.2000000000496,124.723356175805)) ;
#113210=CARTESIAN_POINT('',(-22.3968667215,9.05000000004959,124.757886585629)) ;
#113211=CARTESIAN_POINT('Ctrl Pts',(-22.3968186600187,9.04995061214263,
124.75789795486)) ;
#113212=CARTESIAN_POINT('Ctrl Pts',(-22.5428381268374,9.2000000000496,124.723356175805)) ;
#113213=CARTESIAN_POINT('Ctrl Pts',(-22.0524359330944,9.04995061214263,
123.301650939299)) ;
#113214=CARTESIAN_POINT('Ctrl Pts',(-22.1962101373909,9.2000000000496,123.257614912411)) ;
#113215=CARTESIAN_POINT('Ctrl Pts',(-21.5654953531972,9.04995061214263,
121.879169191031)) ;
#113216=CARTESIAN_POINT('Ctrl Pts',(-21.7060948744266,9.2000000000496,121.82585907834)) ;
#113217=CARTESIAN_POINT('Ctrl Pts',(-20.9452106020614,9.04995061214263,
120.517368302317)) ;
#113218=CARTESIAN_POINT('Ctrl Pts',(-21.0817660968248,9.2000000000496,120.455179752781)) ;
#113219=CARTESIAN_POINT('Ctrl Pts',(5.45900038311354,9.0350000000496,134.413702396319)) ;
#113220=CARTESIAN_POINT('Ctrl Pts',(5.58795314825178,9.2000000000496,134.516640166064)) ;
#113221=CARTESIAN_POINT('Ctrl Pts',(4.91174063504482,9.0350000000496,135.099780839932)) ;
#113222=CARTESIAN_POINT('Ctrl Pts',(5.02776600408638,9.2000000000496,135.218925186777)) ;
#113223=CARTESIAN_POINT('Ctrl Pts',(3.49838774780947,9.03500000004959,136.311302165659)) ;
#113224=CARTESIAN_POINT('Ctrl Pts',(3.58102682874936,9.20000000004958,136.459065126737)) ;
#113225=CARTESIAN_POINT('Ctrl Pts',(0.800790222613687,9.03500000004959,
137.193634477665)) ;
#113226=CARTESIAN_POINT('Ctrl Pts',(0.819706526786835,9.2000000000496,137.362239934218)) ;
#113227=CARTESIAN_POINT('Ctrl Pts',(-2.02545194877293,9.03500000004959,
136.931045772719)) ;
#113228=CARTESIAN_POINT('Ctrl Pts',(-2.07329727026273,9.20000000004959,
137.093448346514)) ;
#113229=CARTESIAN_POINT('Ctrl Pts',(-4.46212557757601,9.0350000000496,135.645856502129)) ;
#113230=CARTESIAN_POINT('Ctrl Pts',(-4.56753011885253,9.20000000004959,
135.777900274175)) ;
#113231=CARTESIAN_POINT('Ctrl Pts',(-6.25536991162766,9.0350000000496,133.554470232605)) ;
#113232=CARTESIAN_POINT('Ctrl Pts',(-6.40313455515177,9.2000000000496,133.637111179546)) ;
#113233=CARTESIAN_POINT('Ctrl Pts',(-7.13757414785378,9.0350000000496,130.856768222766)) ;
#113234=CARTESIAN_POINT('Ctrl Pts',(-7.30617826165478,9.20000000004959,
130.875683925058)) ;
#113235=CARTESIAN_POINT('Ctrl Pts',(-6.87511186948821,9.03500000004958,
128.030539259957)) ;
#113236=CARTESIAN_POINT('Ctrl Pts',(-7.03751608684004,9.20000000004958,
127.982693648484)) ;
#113237=CARTESIAN_POINT('Ctrl Pts',(-5.58980088850994,9.03500000004961,
125.593879064238)) ;
#113238=CARTESIAN_POINT('Ctrl Pts',(-5.72184342923753,9.2000000000496,125.488474550351)) ;
#113239=CARTESIAN_POINT('Ctrl Pts',(-3.49852050212872,9.03500000004958,
123.800649955475)) ;
#113240=CARTESIAN_POINT('Ctrl Pts',(-3.5811627186061,9.20000000004957,123.652885698944)) ;
#113241=CARTESIAN_POINT('Ctrl Pts',(-0.800686682415543,9.03500000004961,
122.918385781163)) ;
#113242=CARTESIAN_POINT('Ctrl Pts',(-0.819600541308432,9.2000000000496,
122.749780638574)) ;
#113243=CARTESIAN_POINT('Ctrl Pts',(2.0253883534138,9.03500000004958,123.180951083883)) ;
#113244=CARTESIAN_POINT('Ctrl Pts',(2.07323217291338,9.20000000004958,123.018548271325)) ;
#113245=CARTESIAN_POINT('Ctrl Pts',(4.46216996178487,9.03500000004959,124.466165925497)) ;
#113246=CARTESIAN_POINT('Ctrl Pts',(4.56757555136914,9.20000000004958,124.334122518572)) ;
#113247=CARTESIAN_POINT('Ctrl Pts',(6.25532282093323,9.03500000004959,126.557507359097)) ;
#113248=CARTESIAN_POINT('Ctrl Pts',(6.4030863521721,9.20000000004959,126.474865718472)) ;
#113249=CARTESIAN_POINT('Ctrl Pts',(7.13764456841352,9.0350000000496,129.255296325887)) ;
#113250=CARTESIAN_POINT('Ctrl Pts',(7.30625034559879,9.20000000004959,129.236381983343)) ;
#113251=CARTESIAN_POINT('Ctrl Pts',(6.87498454206566,9.0350000000496,132.081352928266)) ;
#113252=CARTESIAN_POINT('Ctrl Pts',(7.03738575174059,9.2000000000496,132.129195828704)) ;
#113253=CARTESIAN_POINT('Ctrl Pts',(6.00676094790199,9.0350000000496,133.728021235528)) ;
#113254=CARTESIAN_POINT('Ctrl Pts',(6.14865293878678,9.20000000004959,133.814761812278)) ;
#113255=CARTESIAN_POINT('Ctrl Pts',(5.45900038311354,9.0350000000496,134.413702396319)) ;
#113256=CARTESIAN_POINT('Ctrl Pts',(5.58795314825178,9.2000000000496,134.516640166064)) ;
#113257=CARTESIAN_POINT('',(5.47072336176247,9.05000000004959,134.423060375387)) ;
#113258=CARTESIAN_POINT('Ctrl Pts',(-34.9039592011489,9.04979412703026,
127.731701439515)) ;
#113259=CARTESIAN_POINT('Ctrl Pts',(-34.9976674182864,9.2000000000496,127.849092131696)) ;
#113260=CARTESIAN_POINT('Ctrl Pts',(-35.7782611147991,9.04979412703026,
127.03430818834)) ;
#113261=CARTESIAN_POINT('Ctrl Pts',(-35.885548055222,9.2000000000496,127.140867712464)) ;
#113262=CARTESIAN_POINT('Ctrl Pts',(-36.5298554822976,9.04979412703025,
126.183688247106)) ;
#113263=CARTESIAN_POINT('Ctrl Pts',(-36.648815376531,9.20000000004959,126.277036858917)) ;
#113264=CARTESIAN_POINT('Ctrl Pts',(-37.1142791502663,9.04979412703026,
125.230162926567)) ;
#113265=CARTESIAN_POINT('Ctrl Pts',(-37.2423156796051,9.2000000000496,125.308702418377)) ;
#113266=CARTESIAN_POINT('',(-37.1144546378578,9.05000000004959,125.230270573239)) ;
#113267=CARTESIAN_POINT('',(-34.9976674182864,9.2000000000496,127.849092131696)) ;
#113268=CARTESIAN_POINT('Ctrl Pts',(-37.1082337249472,9.04599943216395,
125.232675075925)) ;
#113269=CARTESIAN_POINT('Ctrl Pts',(-37.2392155304809,9.2000000000496,125.313661591374)) ;
#113270=CARTESIAN_POINT('Ctrl Pts',(-37.3179597355144,9.04599943216395,
124.898605624879)) ;
#113271=CARTESIAN_POINT('Ctrl Pts',(-37.470531050067,9.2000000000496,124.945202526875)) ;
#113272=CARTESIAN_POINT('Ctrl Pts',(-37.4144690154477,9.04599943216395,
124.271498541862)) ;
#113273=CARTESIAN_POINT('Ctrl Pts',(-37.576975151988,9.20000000004958,124.253540041622)) ;
#113274=CARTESIAN_POINT('Ctrl Pts',(-37.0774440110852,9.04599943216397,
123.544161120042)) ;
#113275=CARTESIAN_POINT('Ctrl Pts',(-37.2052562543511,9.20000000004962,
123.451329344491)) ;
#113276=CARTESIAN_POINT('Ctrl Pts',(-36.6386902271357,9.04599943216393,
123.13739949304)) ;
#113277=CARTESIAN_POINT('Ctrl Pts',(-36.7213364569814,9.20000000004957,
123.002695027438)) ;
#113278=CARTESIAN_POINT('Ctrl Pts',(-36.0767657044606,9.04599943216394,
122.930336957724)) ;
#113279=CARTESIAN_POINT('Ctrl Pts',(-36.1015665274975,9.20000000004959,
122.774317144308)) ;
#113280=CARTESIAN_POINT('Ctrl Pts',(-35.276205492832,9.04599943216394,122.95988896865)) ;
#113281=CARTESIAN_POINT('Ctrl Pts',(-35.2185953694054,9.20000000004958,
122.806911285417)) ;
#113282=CARTESIAN_POINT('Ctrl Pts',(-34.7604852661333,9.04599943216395,
123.329749691522)) ;
#113283=CARTESIAN_POINT('Ctrl Pts',(-34.6497860829949,9.20000000004959,
123.214846063503)) ;
#113284=CARTESIAN_POINT('Ctrl Pts',(-34.5579126235981,9.04599943216395,
123.668270050405)) ;
#113285=CARTESIAN_POINT('Ctrl Pts',(-34.426360247948,9.2000000000496,123.588214307529)) ;
#113286=CARTESIAN_POINT('',(-34.557234512772,9.05000000004959,123.661632554657)) ;
#113287=CARTESIAN_POINT('Ctrl Pts',(-34.557234512772,9.05000000004959,123.661632554657)) ;
#113288=CARTESIAN_POINT('Ctrl Pts',(-34.4293734856409,9.2000000000496,123.583200684669)) ;
#113289=CARTESIAN_POINT('Ctrl Pts',(-34.1540823463917,9.05000000004959,
124.319401976811)) ;
#113290=CARTESIAN_POINT('Ctrl Pts',(-34.0352854825652,9.20000000004958,
124.226181328024)) ;
#113291=CARTESIAN_POINT('Ctrl Pts',(-33.6356107525321,9.0500000000496,124.906184432313)) ;
#113292=CARTESIAN_POINT('Ctrl Pts',(-33.528470849969,9.2000000000496,124.799770967498)) ;
#113293=CARTESIAN_POINT('Ctrl Pts',(-33.0324919366153,9.05000000004959,
125.387266520802)) ;
#113294=CARTESIAN_POINT('Ctrl Pts',(-32.9389121460902,9.2000000000496,125.270036734502)) ;
#113295=CARTESIAN_POINT('',(-32.9389121458628,9.2000000000496,125.270036734223)) ;
#113296=CARTESIAN_POINT('Ctrl Pts',(-33.0324919366153,9.05000000004959,
125.387266520802)) ;
#113297=CARTESIAN_POINT('Ctrl Pts',(-32.9389121456355,9.2000000000496,125.270036733944)) ;
#113298=CARTESIAN_POINT('Ctrl Pts',(-32.7232141786936,9.05000000004961,
125.630844357562)) ;
#113299=CARTESIAN_POINT('Ctrl Pts',(-32.5987066128391,9.2000000000496,125.537972355178)) ;
#113300=CARTESIAN_POINT('Ctrl Pts',(-32.4204160994068,9.05000000004959,
126.18773162192)) ;
#113301=CARTESIAN_POINT('Ctrl Pts',(-32.2656287248248,9.2000000000496,126.150548345613)) ;
#113302=CARTESIAN_POINT('Ctrl Pts',(-32.4901171834901,9.0500000000496,126.9866625619)) ;
#113303=CARTESIAN_POINT('Ctrl Pts',(-32.3422999176508,9.2000000000496,127.029372379786)) ;
#113304=CARTESIAN_POINT('Ctrl Pts',(-32.7651801374046,9.0500000000496,127.51978310261)) ;
#113305=CARTESIAN_POINT('Ctrl Pts',(-32.6448691671967,9.2000000000496,127.615804974768)) ;
#113306=CARTESIAN_POINT('Ctrl Pts',(-33.2244615084222,9.0500000000496,127.906584773892)) ;
#113307=CARTESIAN_POINT('Ctrl Pts',(-33.1500786747586,9.2000000000496,128.041286812588)) ;
#113308=CARTESIAN_POINT('Ctrl Pts',(-33.9877047687723,9.0500000000496,128.151068223783)) ;
#113309=CARTESIAN_POINT('Ctrl Pts',(-33.9896462617629,9.2000000000496,128.310218608482)) ;
#113310=CARTESIAN_POINT('Ctrl Pts',(-34.5981365140358,9.0500000000496,127.979692383621)) ;
#113311=CARTESIAN_POINT('Ctrl Pts',(-34.6611211806255,9.20000000004961,
128.121705182437)) ;
#113312=CARTESIAN_POINT('Ctrl Pts',(-34.9040876381615,9.05000000004959,
127.731862335862)) ;
#113313=CARTESIAN_POINT('Ctrl Pts',(-34.9976674182864,9.2000000000496,127.849092131696)) ;
#196737=UNCERTAINTY_MEASURE_WITH_UNIT(LENGTH_MEASURE(0.01),#196742,
'DISTANCE_ACCURACY_VALUE',
'Maximum model space distance between geometric entities at asserted c
onnectivities') ;
#196738=UNCERTAINTY_MEASURE_WITH_UNIT(LENGTH_MEASURE(0.01),#196742,
'DISTANCE_ACCURACY_VALUE',
'Maximum model space distance between geometric entities at asserted c
onnectivities') ;
#196740=(
GEOMETRIC_REPRESENTATION_CONTEXT(3)
GLOBAL_UNCERTAINTY_ASSIGNED_CONTEXT((#196737))
GLOBAL_UNIT_ASSIGNED_CONTEXT((#196742,#196744,#196745))
REPRESENTATION_CONTEXT('','3D')
) ;
#196741=(
GEOMETRIC_REPRESENTATION_CONTEXT(3)
GLOBAL_UNCERTAINTY_ASSIGNED_CONTEXT((#196738))
GLOBAL_UNIT_ASSIGNED_CONTEXT((#196742,#196744,#196745))
REPRESENTATION_CONTEXT('','3D')
) ;
#196742=(
LENGTH_UNIT()
NAMED_UNIT(*)
SI_UNIT(.MILLI.,.METRE.)
) ;
#196744=(
NAMED_UNIT(*)
PLANE_ANGLE_UNIT()
SI_UNIT($,.RADIAN.)
) ;
#196745=(
NAMED_UNIT(*)
SI_UNIT($,.STERADIAN.)
SOLID_ANGLE_UNIT()
) ;
#196753=PRODUCT_DEFINITION_CONTEXT('part definition',#196761,'design') ;
#196761=APPLICATION_CONTEXT(
'Core Data for Automotive Mechanical Design Process') ;
#196762=PRODUCT_CONTEXT('part definition',#196761,'mechanical') ;
#196765=PRESENTATION_STYLE_ASSIGNMENT((#196767)) ;
#196767=SURFACE_STYLE_USAGE(.BOTH.,#196769) ;
#196769=SURFACE_SIDE_STYLE('',(#196771)) ;
#196771=SURFACE_STYLE_FILL_AREA(#196773) ;
#196773=FILL_AREA_STYLE('Steel - Satin',(#196775)) ;
#196775=FILL_AREA_STYLE_COLOUR('Steel - Satin',#196777) ;
#196777=COLOUR_RGB('Steel - Satin', 0.09019608, 0.27058824, 0.51372549) ;
#196923=CARTESIAN_POINT ( '', ( 0.0, 0.0, 0.0 ) ) ;
#196924=DIRECTION ( '', ( 0.0, 0.0, 1.0 ) ) ;
#196925=DIRECTION ( '', ( 1.0, 0.0, 0.0 ) ) ;
#196926=AXIS2_PLACEMENT_3D ( '', #196923, #196924, #196925 ) ;
#196927=ADVANCED_BREP_SHAPE_REPRESENTATION ( 'Entry Pallet Arm', ( #344, #196926, #196937, #197316 ), #196740 ) ;
#196928=PRODUCT( 'Entry Pallet Arm', 'Entry Pallet Arm', '', ( #196762 ) ) ;
#196929=PRODUCT_DEFINITION_FORMATION ( '', '', #196928 ) ;
#196930=PRODUCT_DEFINITION( 'Entry Pallet Arm', 'Entry Pallet Arm', #196929, #196753 ) ;
#196931=PRODUCT_DEFINITION_SHAPE ( '', '', #196930 ) ;
#196932=SHAPE_DEFINITION_REPRESENTATION ( #196931, #196927 ) ;
#196934=CARTESIAN_POINT ( '', ( 0.0, 0.0, 0.0 ) ) ;
#196935=DIRECTION ( '', ( 0.0, 0.0, 1.0 ) ) ;
#196936=DIRECTION ( '', ( 1.0, 0.0, 0.0 ) ) ;
#196937=AXIS2_PLACEMENT_3D ( '', #196934, #196935, #196936 ) ;
#197313=CARTESIAN_POINT ( '', ( 0.0, 0.0, 0.0 ) ) ;
#197314=DIRECTION ( '', ( 0.0, 0.0, 1.0 ) ) ;
#197315=DIRECTION ( '', ( 1.0, 0.0, 0.0 ) ) ;
#197316=AXIS2_PLACEMENT_3D ( '', #197313, #197314, #197315 ) ;
ENDSEC;
END-ISO-10303-21;
